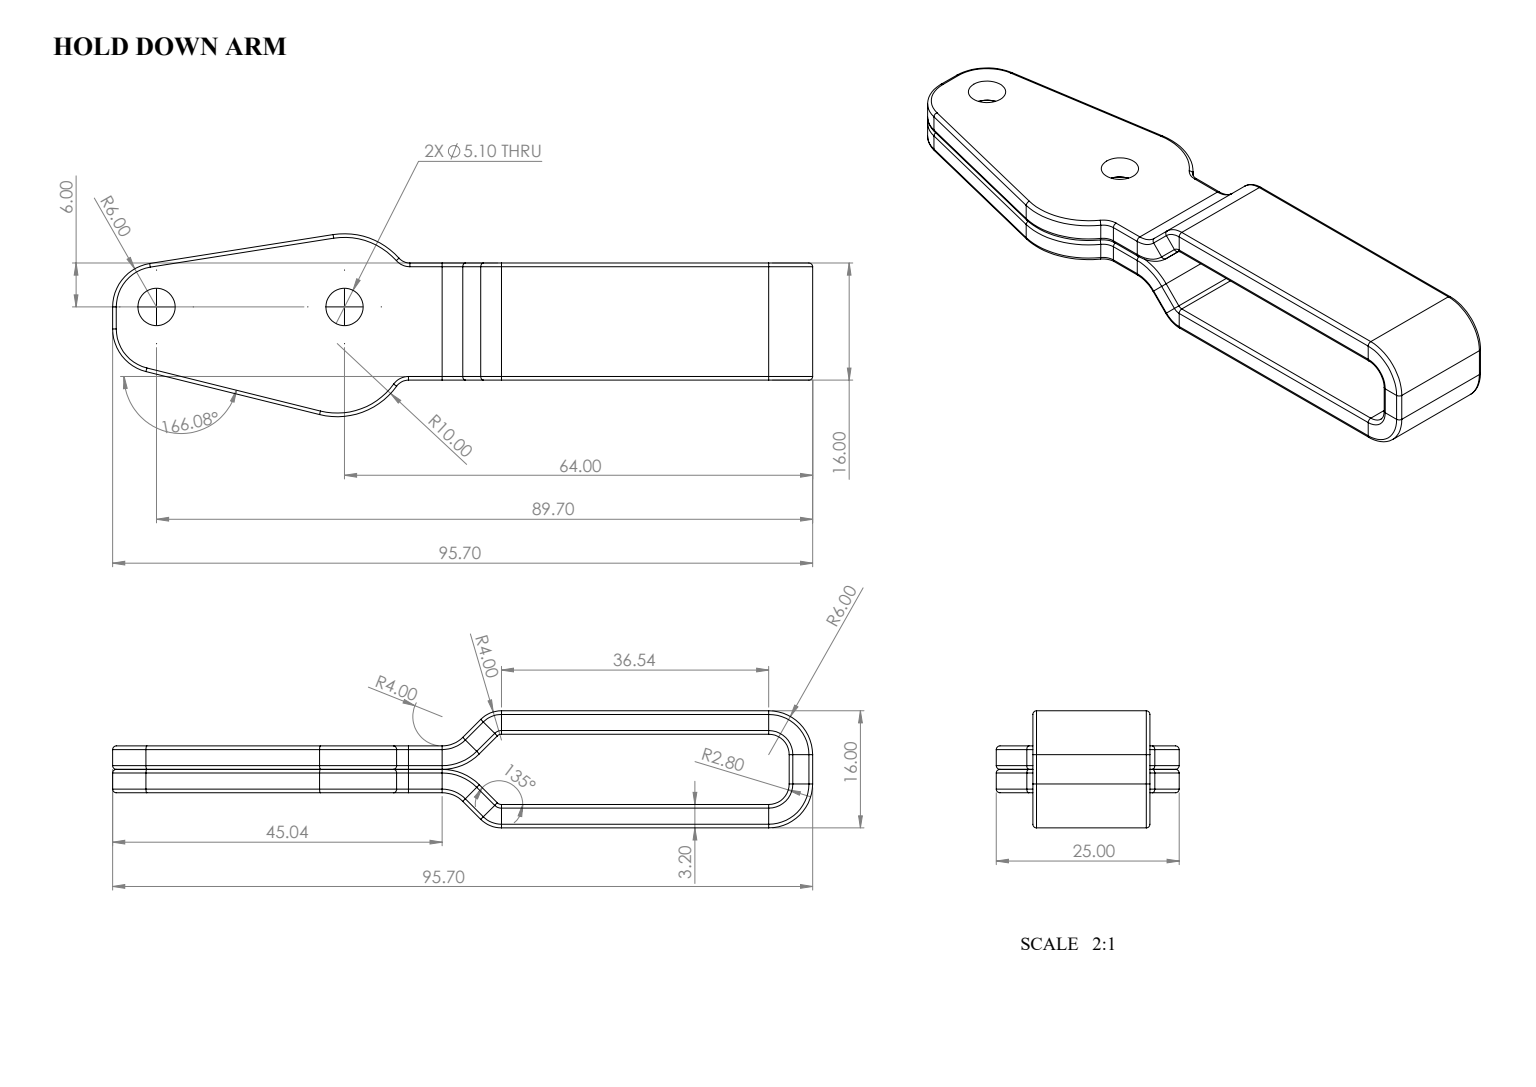
ISO-10303-21;
HEADER;
FILE_DESCRIPTION (('STEP AP214'),
    '1' );
FILE_NAME ('Hold Down Arm.step',
    '2026-10-06T08:09:25',
    ( '' ),
    ( '' ),
    'SwSTEP 2.0',
    'SolidWorks 2021',
    '' );
FILE_SCHEMA (( 'AUTOMOTIVE_DESIGN' ));
ENDSEC;

DATA;
#4=ORIENTED_EDGE ( 'NONE', *, *, #13581, .T. ) ;
#8=DIRECTION ( 'NONE',  ( 1.000000000000000000, 2.220446049250314560E-16, 0.000000000000000000 ) ) ;
#9=CARTESIAN_POINT ( 'NONE',  ( -55.05572809000119605, -2.700000000000125855, -7.500000000000062172 ) ) ;
#14=EDGE_LOOP ( 'NONE', ( #2614, #10567, #22264, #5073 ) ) ;
#18=DIRECTION ( 'NONE',  ( -1.000000000000000000, 1.424116703980815236E-16, 2.931272055834072749E-32 ) ) ;
#20=CARTESIAN_POINT ( 'NONE',  ( -47.82842712474649716, 4.371572875253824542, 8.000000000000021316 ) ) ;
#27=CARTESIAN_POINT ( 'NONE',  ( -50.65685424949274562, -3.200000000000091660, 7.500000000000076383 ) ) ;
#30=ORIENTED_EDGE ( 'NONE', *, *, #19301, .F. ) ;
#33=ORIENTED_EDGE ( 'NONE', *, *, #6783, .T. ) ;
#46=FACE_OUTER_BOUND ( 'NONE', #18970, .T. ) ;
#63=ORIENTED_EDGE ( 'NONE', *, *, #11679, .F. ) ;
#66=ORIENTED_EDGE ( 'NONE', *, *, #4342, .F. ) ;
#67=EDGE_CURVE ( 'NONE', #21664, #15682, #5815, .T. ) ;
#70=CARTESIAN_POINT ( 'NONE',  ( -42.54314575050785407, -5.300000000000037126, -7.500000000000007105 ) ) ;
#73=DIRECTION ( 'NONE',  ( -0.9878135252003118483, -1.627025617018325989E-30, 0.1556420233463095271 ) ) ;
#78=EDGE_CURVE ( 'NONE', #1099, #6825, #11430, .T. ) ;
#91=CIRCLE ( 'NONE', #20737, 0.4999999999999994449 ) ;
#92=ORIENTED_EDGE ( 'NONE', *, *, #20127, .T. ) ;
#96=DIRECTION ( 'NONE',  ( -4.336808689942052446E-15, -1.000000000000000000, -3.574525976782710619E-31 ) ) ;
#98=DIRECTION ( 'NONE',  ( 0.000000000000000000, -1.000000000000000000, 0.000000000000000000 ) ) ;
#99=DIRECTION ( 'NONE',  ( -1.000000000000000000, -2.220446049250313081E-16, 0.000000000000000000 ) ) ;
#101=ADVANCED_FACE ( 'NONE', ( #18737 ), #22509, .T. ) ;
#103=DIRECTION ( 'NONE',  ( -2.220446049250313081E-16, 1.000000000000000000, -7.025792437124636392E-31 ) ) ;
#105=LINE ( 'NONE', #16189, #2754 ) ;
#118=AXIS2_PLACEMENT_3D ( 'NONE', #12279, #12167, #17943 ) ;
#119=DIRECTION ( 'NONE',  ( -1.000000000000000000, -1.479114197289388027E-30, 2.013525853228518840E-32 ) ) ;
#121=AXIS2_PLACEMENT_3D ( 'NONE', #9275, #21645, #19978 ) ;
#122=CARTESIAN_POINT ( 'NONE',  ( -92.25000000000058265, -8.981013850637800498E-14, -2.000000000000001776 ) ) ;
#126=DIRECTION ( 'NONE',  ( 2.013525853228507892E-32, 6.902532920683810383E-31, -1.000000000000000000 ) ) ;
#128=CARTESIAN_POINT ( 'NONE',  ( -89.70000000000064233, 2.700000000000056577, -2.000000000000001776 ) ) ;
#131=CYLINDRICAL_SURFACE ( 'NONE', #16076, 2.000000000000015543 ) ;
#137=AXIS2_PLACEMENT_3D ( 'NONE', #8620, #22982, #10500 ) ;
#139=AXIS2_PLACEMENT_3D ( 'NONE', #3664, #23097, #6847 ) ;
#152=AXIS2_PLACEMENT_3D ( 'NONE', #5181, #12341, #17885 ) ;
#154=TOROIDAL_SURFACE ( 'NONE', #10279, 5.500000000000007994, 0.5000000000000000000 ) ;
#155=CARTESIAN_POINT ( 'NONE',  ( -55.25320565519145788, 0.5000000000000905942, 10.00000000000009237 ) ) ;
#156=VECTOR ( 'NONE', #8671, 1000.000000000000227 ) ;
#158=AXIS2_PLACEMENT_3D ( 'NONE', #22123, #20356, #13067 ) ;
#160=DIRECTION ( 'NONE',  ( 1.000000000000000000, 2.220446049250313081E-16, -3.656342123407315983E-48 ) ) ;
#170=AXIS2_PLACEMENT_3D ( 'NONE', #22281, #4382, #9585 ) ;
#173=VECTOR ( 'NONE', #16606, 1000.000000000000000 ) ;
#183=EDGE_CURVE ( 'NONE', #9368, #15940, #10370, .T. ) ;
#184=EDGE_CURVE ( 'NONE', #21240, #19103, #1689, .T. ) ;
#185=FACE_OUTER_BOUND ( 'NONE', #9063, .T. ) ;
#189=FACE_OUTER_BOUND ( 'NONE', #10029, .T. ) ;
#190=CARTESIAN_POINT ( 'NONE',  ( -42.54314575050778302, -8.000000000000021316, 7.500000000000034639 ) ) ;
#196=EDGE_CURVE ( 'NONE', #1099, #11721, #4693, .T. ) ;
#197=EDGE_CURVE ( 'NONE', #5639, #7574, #985, .T. ) ;
#201=AXIS2_PLACEMENT_3D ( 'NONE', #19066, #17054, #16931 ) ;
#218=AXIS2_PLACEMENT_3D ( 'NONE', #14602, #2245, #20126 ) ;
#220=DIRECTION ( 'NONE',  ( -1.000000000000000000, -2.220446049250314067E-16, 5.825996348268307008E-33 ) ) ;
#225=ORIENTED_EDGE ( 'NONE', *, *, #17691, .F. ) ;
#227=EDGE_CURVE ( 'NONE', #18640, #22996, #18594, .T. ) ;
#228=CARTESIAN_POINT ( 'NONE',  ( -55.05572809000122447, -2.700000000000125855, -10.00000000000006395 ) ) ;
#240=DIRECTION ( 'NONE',  ( -2.013525853228508439E-32, -6.779273404243028164E-31, 1.000000000000000000 ) ) ;
#242=DIRECTION ( 'NONE',  ( 1.000000000000000000, 1.479114197289387852E-30, -2.013525853228518840E-32 ) ) ;
#257=FACE_OUTER_BOUND ( 'NONE', #3493, .T. ) ;
#259=FACE_OUTER_BOUND ( 'NONE', #10192, .T. ) ;
#274=ORIENTED_EDGE ( 'NONE', *, *, #19427, .F. ) ;
#276=EDGE_LOOP ( 'NONE', ( #1805, #8526, #7103, #1700 ) ) ;
#278=VERTEX_POINT ( 'NONE', #17790 ) ;
#292=DIRECTION ( 'NONE',  ( 0.7071067811865535679, -0.7071067811865414665, 0.000000000000000000 ) ) ;
#298=CARTESIAN_POINT ( 'NONE',  ( -56.87767137932624451, -2.700000000000049472, 8.833333333333415638 ) ) ;
#302=ORIENTED_EDGE ( 'NONE', *, *, #6662, .T. ) ;
#305=CARTESIAN_POINT ( 'NONE',  ( -90.55603112840523750, -3.200000000000105427, -7.432974388601742533 ) ) ;
#307=ORIENTED_EDGE ( 'NONE', *, *, #10358, .F. ) ;
#309=ORIENTED_EDGE ( 'NONE', *, *, #10119, .F. ) ;
#310=AXIS2_PLACEMENT_3D ( 'NONE', #22356, #6236, #2234 ) ;
#311=ORIENTED_EDGE ( 'NONE', *, *, #11203, .F. ) ;
#316=LINE ( 'NONE', #16179, #14360 ) ;
#319=FACE_OUTER_BOUND ( 'NONE', #20806, .T. ) ;
#326=DIRECTION ( 'NONE',  ( 1.000000000000000000, 2.220446049250314067E-16, -5.825996348268307008E-33 ) ) ;
#329=CIRCLE ( 'NONE', #8202, 0.5000000000000004441 ) ;
#332=DIRECTION ( 'NONE',  ( 1.550910762415513985E-16, 1.000000000000000000, -8.135128085091684243E-31 ) ) ;
#333=EDGE_CURVE ( 'NONE', #15092, #15826, #3886, .T. ) ;
#336=EDGE_CURVE ( 'NONE', #17272, #9446, #19746, .T. ) ;
#369=PRODUCT_CONTEXT ( 'NONE', #23224, 'mechanical' ) ;
#377=DIRECTION ( 'NONE',  ( 0.2405376366294273427, 0.000000000000000000, -0.9706398123736372785 ) ) ;
#391=CARTESIAN_POINT ( 'NONE',  ( -0.5000000000000559552, -1.999999999999988010, -8.000000000000062172 ) ) ;
#394=EDGE_LOOP ( 'NONE', ( #15847, #9130, #15878, #21668 ) ) ;
#395=ORIENTED_EDGE ( 'NONE', *, *, #6942, .F. ) ;
#400=EDGE_LOOP ( 'NONE', ( #7462, #10799, #18667, #12854 ) ) ;
#409=DIRECTION ( 'NONE',  ( -2.220446049250313081E-16, 1.000000000000000000, -7.025792437124636392E-31 ) ) ;
#416=DIRECTION ( 'NONE',  ( 1.000000000000000000, 6.640738306473676004E-15, 4.078150875473213127E-31 ) ) ;
#425=ORIENTED_EDGE ( 'NONE', *, *, #22642, .T. ) ;
#426=EDGE_CURVE ( 'NONE', #22532, #14335, #5472, .T. ) ;
#436=CARTESIAN_POINT ( 'NONE',  ( -91.14322581977729953, 0.5000000000000073275, 6.823838874241844543 ) ) ;
#441=( LENGTH_UNIT ( ) NAMED_UNIT ( * ) SI_UNIT ( .MILLI., .METRE. ) );
#442=DIRECTION ( 'NONE',  ( -1.550910762415566494E-16, -1.000000000000000000, 8.135128085091684243E-31 ) ) ;
#454=CARTESIAN_POINT ( 'NONE',  ( -43.10883117545721888, 4.565685424949256443, -7.500000000000034639 ) ) ;
#455=FACE_OUTER_BOUND ( 'NONE', #14770, .T. ) ;
#460=CARTESIAN_POINT ( 'NONE',  ( -89.70000000000065654, 3.200000000000057021, -2.000000000000001776 ) ) ;
#461=EDGE_CURVE ( 'NONE', #6874, #3000, #20486, .T. ) ;
#472=EDGE_CURVE ( 'NONE', #1433, #3000, #8099, .T. ) ;
#474=EDGE_CURVE ( 'NONE', #5438, #4432, #6471, .T. ) ;
#477=VERTEX_POINT ( 'NONE', #15401 ) ;
#484=EDGE_CURVE ( 'NONE', #1099, #2832, #13652, .T. ) ;
#487=CYLINDRICAL_SURFACE ( 'NONE', #2237, 0.5000000000000029976 ) ;
#489=ORIENTED_EDGE ( 'NONE', *, *, #12121, .F. ) ;
#490=PLANE ( 'NONE',  #19494 ) ;
#498=CIRCLE ( 'NONE', #14398, 0.4999999999999994449 ) ;
#506=CARTESIAN_POINT ( 'NONE',  ( -42.54314575050799618, 4.799999999999998934, 8.000000000000035527 ) ) ;
#510=ORIENTED_EDGE ( 'NONE', *, *, #22197, .F. ) ;
#511=ORIENTED_EDGE ( 'NONE', *, *, #15896, .T. ) ;
#512=ORIENTED_EDGE ( 'NONE', *, *, #15274, .F. ) ;
#521=AXIS2_PLACEMENT_3D ( 'NONE', #8817, #5413, #15970 ) ;
#529=FACE_OUTER_BOUND ( 'NONE', #12268, .T. ) ;
#535=CARTESIAN_POINT ( 'NONE',  ( -89.70000000000054285, -9.020562075079396891E-14, 1.000000000000000888 ) ) ;
#544=EDGE_LOOP ( 'NONE', ( #3998, #20221, #14255, #14599 ) ) ;
#549=ADVANCED_FACE ( 'NONE', ( #5291 ), #15517, .T. ) ;
#553=AXIS2_PLACEMENT_3D ( 'NONE', #6003, #7641, #3986 ) ;
#554=FACE_OUTER_BOUND ( 'NONE', #6636, .T. ) ;
#557=EDGE_CURVE ( 'NONE', #19870, #14824, #11076, .T. ) ;
#559=CARTESIAN_POINT ( 'NONE',  ( -42.54314575050781144, -3.999999999999996447, -16.42537846091818210 ) ) ;
#565=CARTESIAN_POINT ( 'NONE',  ( -50.65685424949274562, -3.200000000000091660, 8.000000000000062172 ) ) ;
#571=ORIENTED_EDGE ( 'NONE', *, *, #22014, .F. ) ;
#576=CARTESIAN_POINT ( 'NONE',  ( -6.000000000000199840, 4.799999999999935874, 8.000000000000035527 ) ) ;
#578=DIRECTION ( 'NONE',  ( 0.7071067811865510144, 0.7071067811865441310, -9.779905552809737959E-15 ) ) ;
#586=EDGE_CURVE ( 'NONE', #15196, #6243, #21185, .T. ) ;
#600=CIRCLE ( 'NONE', #8864, 0.5000000000000028866 ) ;
#607=DIRECTION ( 'NONE',  ( 0.7071067811865502373, -0.7071067811865447972, -5.485661035786110830E-15 ) ) ;
#608=DIRECTION ( 'NONE',  ( 0.2405376366294550983, 0.000000000000000000, -0.9706398123736303951 ) ) ;
#630=ORIENTED_EDGE ( 'NONE', *, *, #14353, .F. ) ;
#653=EDGE_CURVE ( 'NONE', #19930, #15092, #3743, .T. ) ;
#658=ORIENTED_EDGE ( 'NONE', *, *, #15288, .F. ) ;
#665=AXIS2_PLACEMENT_3D ( 'NONE', #19621, #7167, #5157 ) ;
#668=CYLINDRICAL_SURFACE ( 'NONE', #15478, 0.5000000000000004441 ) ;
#671=VECTOR ( 'NONE', #10328, 1000.000000000000227 ) ;
#680=FACE_OUTER_BOUND ( 'NONE', #17185, .T. ) ;
#684=PLANE ( 'NONE',  #18357 ) ;
#691=ORIENTED_EDGE ( 'NONE', *, *, #20005, .F. ) ;
#713=CARTESIAN_POINT ( 'NONE',  ( -50.65685424949278826, 1.387778780781445676E-14, -7.500000000000034639 ) ) ;
#718=ORIENTED_EDGE ( 'NONE', *, *, #16718, .F. ) ;
#748=ORIENTED_EDGE ( 'NONE', *, *, #11622, .T. ) ;
#751=CARTESIAN_POINT ( 'NONE',  ( -49.51923881554282048, 1.137615433949801247, 7.500000000000062172 ) ) ;
#752=EDGE_CURVE ( 'NONE', #15489, #3212, #12450, .T. ) ;
#755=AXIS2_PLACEMENT_3D ( 'NONE', #13105, #409, #21706 ) ;
#756=DIRECTION ( 'NONE',  ( -1.000000000000000000, -1.479114197289388027E-30, 2.013525853228518840E-32 ) ) ;
#761=EDGE_CURVE ( 'NONE', #18638, #13378, #23145, .T. ) ;
#764=EDGE_CURVE ( 'NONE', #8174, #11574, #3261, .T. ) ;
#768=CARTESIAN_POINT ( 'NONE',  ( -95.20000000000061391, -0.5000000000000975886, 8.000000000000117240 ) ) ;
#779=EDGE_CURVE ( 'NONE', #4281, #1775, #20143, .T. ) ;
#781=ORIENTED_EDGE ( 'NONE', *, *, #14027, .T. ) ;
#786=ORIENTED_EDGE ( 'NONE', *, *, #13748, .F. ) ;
#787=DIRECTION ( 'NONE',  ( 1.000000000000000000, 1.424116703980846297E-16, -1.095779650622964657E-32 ) ) ;
#789=DIRECTION ( 'NONE',  ( 0.000000000000000000, 0.000000000000000000, 1.000000000000000000 ) ) ;
#792=DIRECTION ( 'NONE',  ( 0.9706398123736330597, 1.110223024625160485E-16, 0.2405376366294442736 ) ) ;
#798=DIRECTION ( 'NONE',  ( 1.000000000000000000, 1.479114197289387852E-30, -2.013525853228518840E-32 ) ) ;
#804=ORIENTED_EDGE ( 'NONE', *, *, #20468, .F. ) ;
#805=ORIENTED_EDGE ( 'NONE', *, *, #9969, .T. ) ;
#812=FACE_OUTER_BOUND ( 'NONE', #7748, .T. ) ;
#813=CARTESIAN_POINT ( 'NONE',  ( -45.91923881554279774, 2.462384566050190848, -7.500000000000062172 ) ) ;
#814=CARTESIAN_POINT ( 'NONE',  ( -89.70000000000057128, -0.5000000000000628386, -2.000000000000001776 ) ) ;
#817=EDGE_CURVE ( 'NONE', #5639, #8174, #15026, .T. ) ;
#830=AXIS2_PLACEMENT_3D ( 'NONE', #9486, #8070, #792 ) ;
#836=CARTESIAN_POINT ( 'NONE',  ( -95.70000000000062812, -1.318389841742373392E-13, 8.000000000000062172 ) ) ;
#837=CARTESIAN_POINT ( 'NONE',  ( -45.37157287525414517, -6.828427124746218269, 7.500000000000089706 ) ) ;
#851=CYLINDRICAL_SURFACE ( 'NONE', #5151, 0.5000000000000000000 ) ;
#852=AXIS2_PLACEMENT_3D ( 'NONE', #14679, #3854, #11035 ) ;
#853=TOROIDAL_SURFACE ( 'NONE', #8348, 3.500000000000000888, 0.5000000000000000000 ) ;
#854=EDGE_LOOP ( 'NONE', ( #1944, #11607, #22757, #20845 ) ) ;
#870=CIRCLE ( 'NONE', #1976, 0.5000000000000004441 ) ;
#873=CARTESIAN_POINT ( 'NONE',  ( -50.65685424949273141, 0.000000000000000000, 8.000000000000076383 ) ) ;
#876=( NAMED_UNIT ( * ) PLANE_ANGLE_UNIT ( ) SI_UNIT ( $, .RADIAN. ) );
#881=DIRECTION ( 'NONE',  ( -0.9878135252003118483, -1.627025617018325989E-30, 0.1556420233463091385 ) ) ;
#883=EDGE_CURVE ( 'NONE', #16517, #14933, #8878, .T. ) ;
#885=AXIS2_PLACEMENT_3D ( 'NONE', #5509, #21519, #6803 ) ;
#890=AXIS2_PLACEMENT_3D ( 'NONE', #12840, #9317, #16129 ) ;
#893=AXIS2_PLACEMENT_3D ( 'NONE', #20867, #8852, #2976 ) ;
#899=ORIENTED_EDGE ( 'NONE', *, *, #5134, .F. ) ;
#901=DIRECTION ( 'NONE',  ( 2.013525853228507892E-32, 6.902532920683810383E-31, -1.000000000000000000 ) ) ;
#929=ORIENTED_EDGE ( 'NONE', *, *, #11228, .T. ) ;
#936=DIRECTION ( 'NONE',  ( 4.336808689942052446E-15, 1.000000000000000000, 3.574525976782710619E-31 ) ) ;
#937=DIRECTION ( 'NONE',  ( 1.000000000000000000, -1.389842848855773367E-62, 2.013525853228507892E-32 ) ) ;
#939=DIRECTION ( 'NONE',  ( -1.000000000000000000, 1.550910762415508562E-16, 0.000000000000000000 ) ) ;
#943=EDGE_CURVE ( 'NONE', #17067, #4165, #11494, .T. ) ;
#959=DIRECTION ( 'NONE',  ( 1.331202777560457422E-30, 1.000000000000000000, -7.395570986446985676E-31 ) ) ;
#964=DIRECTION ( 'NONE',  ( -1.550910762415566494E-16, -1.000000000000000000, 8.135128085091684243E-31 ) ) ;
#972=FACE_OUTER_BOUND ( 'NONE', #13994, .T. ) ;
#985=LINE ( 'NONE', #6982, #17847 ) ;
#988=FACE_OUTER_BOUND ( 'NONE', #14105, .T. ) ;
#990=CARTESIAN_POINT ( 'NONE',  ( -50.65685424949267457, -7.200000000000049916, 7.500000000000047962 ) ) ;
#997=TOROIDAL_SURFACE ( 'NONE', #5495, 3.500000000000000888, 0.5000000000000000000 ) ;
#1001=CARTESIAN_POINT ( 'NONE',  ( -6.000000000000074607, -8.000000000000003553, -7.500000000000034639 ) ) ;
#1006=ORIENTED_EDGE ( 'NONE', *, *, #15901, .F. ) ;
#1014=CARTESIAN_POINT ( 'NONE',  ( -50.65685424949281668, 3.200000000000022382, 7.500000000000034639 ) ) ;
#1015=ORIENTED_EDGE ( 'NONE', *, *, #15615, .T. ) ;
#1021=DIRECTION ( 'NONE',  ( 2.220446049250313081E-16, -1.000000000000000000, 7.025792437124636392E-31 ) ) ;
#1030=CIRCLE ( 'NONE', #4015, 0.5000000000000029976 ) ;
#1041=DIRECTION ( 'NONE',  ( 1.550910762415513985E-16, 1.000000000000000000, -8.135128085091684243E-31 ) ) ;
#1051=DIRECTION ( 'NONE',  ( 1.550910762415566494E-16, 1.000000000000000000, -8.135128085091684243E-31 ) ) ;
#1054=CARTESIAN_POINT ( 'NONE',  ( -92.25000000000065370, 5.494493748869900097E-14, -2.000000000000001776 ) ) ;
#1057=CARTESIAN_POINT ( 'NONE',  ( -45.01801948466093961, 6.474873734152897242, -8.000000000000035527 ) ) ;
#1059=ADVANCED_FACE ( 'NONE', ( #812 ), #22427, .T. ) ;
#1062=CARTESIAN_POINT ( 'NONE',  ( -50.65685424949278826, 0.5000000000000213163, -7.500000000000034639 ) ) ;
#1065=AXIS2_PLACEMENT_3D ( 'NONE', #21849, #15010, #2543 ) ;
#1067=ORIENTED_EDGE ( 'NONE', *, *, #6289, .F. ) ;
#1083=STYLED_ITEM ( 'NONE', ( #20322 ), #15045 ) ;
#1088=CARTESIAN_POINT ( 'NONE',  ( -50.65685424949274562, -2.700000000000125855, 7.500000000000076383 ) ) ;
#1092=DIRECTION ( 'NONE',  ( -1.000000000000000000, -1.479114197289388027E-30, 2.013525853228518840E-32 ) ) ;
#1093=AXIS2_PLACEMENT_3D ( 'NONE', #20642, #18858, #1223 ) ;
#1099=VERTEX_POINT ( 'NONE', #13509 ) ;
#1101=EDGE_LOOP ( 'NONE', ( #16948, #7826, #13990, #15195 ) ) ;
#1107=AXIS2_PLACEMENT_3D ( 'NONE', #3565, #5092, #19911 ) ;
#1123=ADVANCED_FACE ( 'NONE', ( #22447 ), #17133, .T. ) ;
#1124=ORIENTED_EDGE ( 'NONE', *, *, #13695, .F. ) ;
#1136=VERTEX_POINT ( 'NONE', #10199 ) ;
#1151=CARTESIAN_POINT ( 'NONE',  ( -55.05572809000119605, -0.5000000000001045830, -8.000000000000090594 ) ) ;
#1152=ORIENTED_EDGE ( 'NONE', *, *, #12772, .F. ) ;
#1172=CARTESIAN_POINT ( 'NONE',  ( -42.54314575050796776, 3.999999999999996447, -8.000000000000035527 ) ) ;
#1180=ADVANCED_FACE ( 'NONE', ( #8796 ), #2504, .T. ) ;
#1182=EDGE_CURVE ( 'NONE', #6492, #18669, #10552, .T. ) ;
#1190=CIRCLE ( 'NONE', #19959, 7.200000000000046363 ) ;
#1191=CARTESIAN_POINT ( 'NONE',  ( -55.05572809000130974, 2.700000000000021938, -8.000000000000035527 ) ) ;
#1194=CARTESIAN_POINT ( 'NONE',  ( -42.54314575050792513, 3.999999999999996447, 16.42537846091821052 ) ) ;
#1204=AXIS2_PLACEMENT_3D ( 'NONE', #813, #11495, #13510 ) ;
#1205=ORIENTED_EDGE ( 'NONE', *, *, #8263, .F. ) ;
#1216=DIRECTION ( 'NONE',  ( -1.000000000000000000, 6.938893903907186568E-15, 0.000000000000000000 ) ) ;
#1220=CARTESIAN_POINT ( 'NONE',  ( -91.14322581977729953, 2.700000000000014833, 6.823838874241844543 ) ) ;
#1223=DIRECTION ( 'NONE',  ( -1.000000000000000000, -1.144237745222090235E-17, 1.939787525279694125E-32 ) ) ;
#1224=VECTOR ( 'NONE', #17612, 1000.000000000000114 ) ;
#1225=DIRECTION ( 'NONE',  ( 0.1556420233463076119, 0.000000000000000000, 0.9878135252003121813 ) ) ;
#1226=AXIS2_PLACEMENT_3D ( 'NONE', #7718, #9254, #20081 ) ;
#1237=EDGE_CURVE ( 'NONE', #4862, #16835, #16732, .T. ) ;
#1239=ORIENTED_EDGE ( 'NONE', *, *, #2920, .T. ) ;
#1240=AXIS2_PLACEMENT_3D ( 'NONE', #7811, #18512, #20522 ) ;
#1241=AXIS2_PLACEMENT_3D ( 'NONE', #1247, #17337, #14055 ) ;
#1242=CIRCLE ( 'NONE', #11361, 0.5000000000000029976 ) ;
#1247=CARTESIAN_POINT ( 'NONE',  ( -42.54314575050785407, -4.000000000000034639, -7.500000000000007105 ) ) ;
#1249=CARTESIAN_POINT ( 'NONE',  ( -50.65685424949263904, -7.200000000000071232, -7.500000000000034639 ) ) ;
#1250=CARTESIAN_POINT ( 'NONE',  ( -1.110223024625156540E-13, -1.999999999999988010, 7.500000000000020428 ) ) ;
#1259=VECTOR ( 'NONE', #901, 1000.000000000000000 ) ;
#1270=ORIENTED_EDGE ( 'NONE', *, *, #20922, .F. ) ;
#1274=AXIS2_PLACEMENT_3D ( 'NONE', #6348, #13400, #4804 ) ;
#1289=FACE_OUTER_BOUND ( 'NONE', #19754, .T. ) ;
#1291=DIRECTION ( 'NONE',  ( -2.013525853228507892E-32, -6.902532920683810383E-31, 1.000000000000000000 ) ) ;
#1292=AXIS2_PLACEMENT_3D ( 'NONE', #17237, #11834, #13607 ) ;
#1301=DIRECTION ( 'NONE',  ( -1.550910762415566494E-16, -1.000000000000000000, 8.135128085091684243E-31 ) ) ;
#1304=AXIS2_PLACEMENT_3D ( 'NONE', #16015, #18033, #160 ) ;
#1307=LINE ( 'NONE', #9688, #8776 ) ;
#1309=CARTESIAN_POINT ( 'NONE',  ( -49.51923881554282048, 1.137615433949801247, 8.000000000000062172 ) ) ;
#1310=CARTESIAN_POINT ( 'NONE',  ( -95.70000000000071338, 2.775557561562891351E-14, 1.000000000000070166 ) ) ;
#1313=ADVANCED_FACE ( 'NONE', ( #988 ), #13453, .T. ) ;
#1314=CARTESIAN_POINT ( 'NONE',  ( -87.15000000000064517, 5.607736497381665307E-14, -2.000000000000001332 ) ) ;
#1318=ADVANCED_FACE ( 'NONE', ( #17075 ), #22512, .F. ) ;
#1320=LINE ( 'NONE', #19072, #6700 ) ;
#1321=EDGE_CURVE ( 'NONE', #5639, #8147, #17136, .T. ) ;
#1329=VERTEX_POINT ( 'NONE', #16847 ) ;
#1333=DIRECTION ( 'NONE',  ( -1.144237745221811361E-17, 1.000000000000000000, -7.025792437124636392E-31 ) ) ;
#1338=CARTESIAN_POINT ( 'NONE',  ( -6.000000000000143885, -2.000000000000043521, -8.000000000000035527 ) ) ;
#1339=EDGE_CURVE ( 'NONE', #8929, #15576, #4500, .T. ) ;
#1346=DIRECTION ( 'NONE',  ( 0.000000000000000000, 0.000000000000000000, -1.000000000000000000 ) ) ;
#1348=DIRECTION ( 'NONE',  ( 2.220446049250313081E-16, -1.000000000000000000, 7.025792437124636392E-31 ) ) ;
#1349=CARTESIAN_POINT ( 'NONE',  ( -50.65685424949274562, 0.5000000000000143219, -8.000000000000062172 ) ) ;
#1352=ORIENTED_EDGE ( 'NONE', *, *, #22036, .T. ) ;
#1355=EDGE_LOOP ( 'NONE', ( #9247, #2066, #15136, #15479 ) ) ;
#1374=EDGE_CURVE ( 'NONE', #6466, #18914, #19429, .T. ) ;
#1382=EDGE_LOOP ( 'NONE', ( #8989, #21213, #23151, #14355 ) ) ;
#1383=ORIENTED_EDGE ( 'NONE', *, *, #22635, .F. ) ;
#1384=ORIENTED_EDGE ( 'NONE', *, *, #18533, .F. ) ;
#1386=LINE ( 'NONE', #22918, #16285 ) ;
#1396=TOROIDAL_SURFACE ( 'NONE', #14920, 1.300000000000000711, 0.5000000000000000000 ) ;
#1401=ORIENTED_EDGE ( 'NONE', *, *, #12037, .T. ) ;
#1402=ORIENTED_EDGE ( 'NONE', *, *, #14002, .F. ) ;
#1414=CARTESIAN_POINT ( 'NONE',  ( -64.00000000000045475, 6.245004513516505540E-14, -1.999999999999974021 ) ) ;
#1415=DIRECTION ( 'NONE',  ( -1.331202777560457422E-30, -1.000000000000000000, 7.395570986446985676E-31 ) ) ;
#1418=CIRCLE ( 'NONE', #13068, 2.550000000000010481 ) ;
#1422=DIRECTION ( 'NONE',  ( -2.013525853228507892E-32, -6.902532920683810383E-31, 1.000000000000000000 ) ) ;
#1424=CARTESIAN_POINT ( 'NONE',  ( -50.65685424949280247, 1.387778780781445676E-14, 8.000000000000090594 ) ) ;
#1428=AXIS2_PLACEMENT_3D ( 'NONE', #13780, #1092, #17412 ) ;
#1433=VERTEX_POINT ( 'NONE', #6398 ) ;
#1442=DIRECTION ( 'NONE',  ( -2.220446049250313081E-16, 1.000000000000000000, -7.025792437124636392E-31 ) ) ;
#1444=VECTOR ( 'NONE', #442, 1000.000000000000000 ) ;
#1454=ORIENTED_EDGE ( 'NONE', *, *, #13692, .F. ) ;
#1456=ORIENTED_EDGE ( 'NONE', *, *, #16684, .T. ) ;
#1458=EDGE_CURVE ( 'NONE', #4755, #10141, #22619, .T. ) ;
#1464=ORIENTED_EDGE ( 'NONE', *, *, #21499, .F. ) ;
#1470=CARTESIAN_POINT ( 'NONE',  ( -64.00000000000038369, -3.200000000000081446, -2.000000000000029310 ) ) ;
#1471=EDGE_CURVE ( 'NONE', #21722, #18197, #11793, .T. ) ;
#1482=AXIS2_PLACEMENT_3D ( 'NONE', #12903, #16644, #3954 ) ;
#1486=ORIENTED_EDGE ( 'NONE', *, *, #426, .F. ) ;
#1490=CARTESIAN_POINT ( 'NONE',  ( -89.70000000000055707, -3.200000000000105427, -1.999999999999946265 ) ) ;
#1506=CARTESIAN_POINT ( 'NONE',  ( -2.700000000000119194, 1.999999999999967137, -8.000000000000007105 ) ) ;
#1508=AXIS2_PLACEMENT_3D ( 'NONE', #5115, #8531, #3590 ) ;
#1519=TOROIDAL_SURFACE ( 'NONE', #21814, 6.700000000000001066, 0.5000000000000000000 ) ;
#1521=ORIENTED_EDGE ( 'NONE', *, *, #13820, .F. ) ;
#1524=EDGE_LOOP ( 'NONE', ( #1663, #9843, #66, #6122 ) ) ;
#1525=ORIENTED_EDGE ( 'NONE', *, *, #5225, .T. ) ;
#1532=FACE_OUTER_BOUND ( 'NONE', #21083, .T. ) ;
#1533=DIRECTION ( 'NONE',  ( 1.000000000000000000, 0.000000000000000000, 0.000000000000000000 ) ) ;
#1539=DIRECTION ( 'NONE',  ( 2.013525853228507892E-32, 6.902532920683810383E-31, -1.000000000000000000 ) ) ;
#1551=CARTESIAN_POINT ( 'NONE',  ( -89.70000000000064233, 5.551115123125782702E-14, -2.000000000000001776 ) ) ;
#1552=DIRECTION ( 'NONE',  ( 1.331202777560457422E-30, 1.000000000000000000, -7.395570986446985676E-31 ) ) ;
#1555=CARTESIAN_POINT ( 'NONE',  ( -47.47487373415324186, 4.018019484660559471, 8.000000000000062172 ) ) ;
#1557=DIRECTION ( 'NONE',  ( -1.550910762415566494E-16, -1.000000000000000000, 8.135128085091684243E-31 ) ) ;
#1564=DIRECTION ( 'NONE',  ( 0.000000000000000000, 0.000000000000000000, 1.000000000000000000 ) ) ;
#1575=AXIS2_PLACEMENT_3D ( 'NONE', #22054, #20406, #22400 ) ;
#1588=CYLINDRICAL_SURFACE ( 'NONE', #22687, 2.550000000000010481 ) ;
#1589=LINE ( 'NONE', #13077, #14723 ) ;
#1595=CYLINDRICAL_SURFACE ( 'NONE', #10383, 0.5000000000000000000 ) ;
#1596=ORIENTED_EDGE ( 'NONE', *, *, #20698, .F. ) ;
#1599=LINE ( 'NONE', #16169, #12664 ) ;
#1603=EDGE_LOOP ( 'NONE', ( #13242, #14531, #7061, #6609 ) ) ;
#1612=DIRECTION ( 'NONE',  ( 1.550910762415566494E-16, 1.000000000000000000, -8.135128085091684243E-31 ) ) ;
#1616=ADVANCED_FACE ( 'NONE', ( #19674 ), #7208, .T. ) ;
#1620=VECTOR ( 'NONE', #8184, 1000.000000000000000 ) ;
#1631=ORIENTED_EDGE ( 'NONE', *, *, #653, .F. ) ;
#1632=EDGE_CURVE ( 'NONE', #15165, #21891, #10736, .T. ) ;
#1635=ORIENTED_EDGE ( 'NONE', *, *, #1374, .F. ) ;
#1641=ORIENTED_EDGE ( 'NONE', *, *, #10677, .T. ) ;
#1645=EDGE_CURVE ( 'NONE', #10770, #2913, #600, .T. ) ;
#1650=DIRECTION ( 'NONE',  ( 2.013525853228508439E-32, 6.779273404243028164E-31, -1.000000000000000000 ) ) ;
#1661=DIRECTION ( 'NONE',  ( 1.000000000000000000, 1.479114197289388027E-30, -2.013525853228518840E-32 ) ) ;
#1663=ORIENTED_EDGE ( 'NONE', *, *, #15877, .T. ) ;
#1672=CARTESIAN_POINT ( 'NONE',  ( -67.28510754798018922, 1.387778780781445676E-14, 12.22107821754958579 ) ) ;
#1682=DIRECTION ( 'NONE',  ( 1.387778780781437314E-14, 0.000000000000000000, -1.000000000000000000 ) ) ;
#1684=DIRECTION ( 'NONE',  ( -2.013525853228507892E-32, -6.902532920683810383E-31, 1.000000000000000000 ) ) ;
#1689=CIRCLE ( 'NONE', #7335, 0.5000000000000019984 ) ;
#1693=EDGE_CURVE ( 'NONE', #10146, #11081, #6719, .T. ) ;
#1694=VERTEX_POINT ( 'NONE', #16697 ) ;
#1700=ORIENTED_EDGE ( 'NONE', *, *, #333, .T. ) ;
#1702=ORIENTED_EDGE ( 'NONE', *, *, #17416, .F. ) ;
#1714=CARTESIAN_POINT ( 'NONE',  ( -50.65685424949262483, -7.200000000000071232, -16.89924331519437928 ) ) ;
#1717=DIRECTION ( 'NONE',  ( 1.000000000000000000, -1.365024226554777796E-62, 2.013525853228508713E-32 ) ) ;
#1719=ORIENTED_EDGE ( 'NONE', *, *, #2803, .T. ) ;
#1728=CYLINDRICAL_SURFACE ( 'NONE', #12093, 0.5000000000000004441 ) ;
#1729=CARTESIAN_POINT ( 'NONE',  ( -50.65685424949281668, 1.387778780781445676E-14, 7.500000000000034639 ) ) ;
#1733=LINE ( 'NONE', #14216, #14846 ) ;
#1736=CARTESIAN_POINT ( 'NONE',  ( -90.63385214007844581, 2.700000000000056577, -7.926881151201908615 ) ) ;
#1738=AXIS2_PLACEMENT_3D ( 'NONE', #18433, #332, #9267 ) ;
#1743=VERTEX_POINT ( 'NONE', #11295 ) ;
#1756=DIRECTION ( 'NONE',  ( 2.013525853228507892E-32, 6.902532920683810383E-31, -1.000000000000000000 ) ) ;
#1757=EDGE_CURVE ( 'NONE', #11721, #1694, #2590, .T. ) ;
#1763=CARTESIAN_POINT ( 'NONE',  ( -64.00000000000045475, 0.5000000000000490719, -1.999999999999974021 ) ) ;
#1766=CARTESIAN_POINT ( 'NONE',  ( -65.00000000000044054, -2.700000000000084110, 2.999999999999947153 ) ) ;
#1767=ADVANCED_FACE ( 'NONE', ( #5897 ), #490, .T. ) ;
#1768=ORIENTED_EDGE ( 'NONE', *, *, #752, .T. ) ;
#1770=EDGE_CURVE ( 'NONE', #7684, #10125, #13996, .T. ) ;
#1771=EDGE_CURVE ( 'NONE', #22415, #2139, #22955, .T. ) ;
#1775=VERTEX_POINT ( 'NONE', #12217 ) ;
#1781=DIRECTION ( 'NONE',  ( -3.469446951953634699E-15, 1.000000000000000000, -4.336808689942038246E-15 ) ) ;
#1783=EDGE_CURVE ( 'NONE', #11087, #21212, #20847, .T. ) ;
#1785=AXIS2_PLACEMENT_3D ( 'NONE', #21770, #12462, #242 ) ;
#1790=CARTESIAN_POINT ( 'NONE',  ( -55.05572809000126711, 0.5000000000000143219, -7.500000000000034639 ) ) ;
#1792=DIRECTION ( 'NONE',  ( -2.013525853228507892E-32, -6.902532920683810383E-31, 1.000000000000000000 ) ) ;
#1794=AXIS2_PLACEMENT_3D ( 'NONE', #17282, #15404, #6475 ) ;
#1801=ORIENTED_EDGE ( 'NONE', *, *, #3375, .T. ) ;
#1803=ORIENTED_EDGE ( 'NONE', *, *, #18662, .T. ) ;
#1805=ORIENTED_EDGE ( 'NONE', *, *, #4040, .F. ) ;
#1810=EDGE_CURVE ( 'NONE', #5384, #15489, #6597, .T. ) ;
#1816=DIRECTION ( 'NONE',  ( 0.7071067811865718866, 0.7071067811865232589, 0.000000000000000000 ) ) ;
#1818=EDGE_CURVE ( 'NONE', #7626, #21952, #22831, .T. ) ;
#1830=CARTESIAN_POINT ( 'NONE',  ( -57.28378781035996070, -2.700000000000049472, 8.541666666666781538 ) ) ;
#1831=ORIENTED_EDGE ( 'NONE', *, *, #764, .T. ) ;
#1841=DIRECTION ( 'NONE',  ( -2.220446049250313081E-16, 1.000000000000000000, -7.025792437124636392E-31 ) ) ;
#1844=DIRECTION ( 'NONE',  ( 0.000000000000000000, -1.000000000000000000, 0.000000000000000000 ) ) ;
#1848=CARTESIAN_POINT ( 'NONE',  ( -47.82842712474641189, -4.371572875253862733, 7.500000000000047962 ) ) ;
#1853=FACE_OUTER_BOUND ( 'NONE', #7005, .T. ) ;
#1866=CARTESIAN_POINT ( 'NONE',  ( -6.000000000000074607, 1.999999999999960032, 7.500000000000062172 ) ) ;
#1868=CARTESIAN_POINT ( 'NONE',  ( -43.10883117545713361, 4.565685424949256443, 8.000000000000035527 ) ) ;
#1869=DIRECTION ( 'NONE',  ( 1.000000000000000000, -1.389842848855773583E-62, 2.013525853228507892E-32 ) ) ;
#1874=DIRECTION ( 'NONE',  ( 0.000000000000000000, 0.000000000000000000, -1.000000000000000000 ) ) ;
#1880=VERTEX_POINT ( 'NONE', #10126 ) ;
#1883=VERTEX_POINT ( 'NONE', #6713 ) ;
#1884=ORIENTED_EDGE ( 'NONE', *, *, #13567, .T. ) ;
#1904=EDGE_CURVE ( 'NONE', #16829, #13948, #12688, .T. ) ;
#1905=DIRECTION ( 'NONE',  ( -0.7071067811865485719, 0.7071067811865464625, 1.010793663541191362E-16 ) ) ;
#1910=VERTEX_POINT ( 'NONE', #1191 ) ;
#1919=VERTEX_POINT ( 'NONE', #6956 ) ;
#1923=FACE_OUTER_BOUND ( 'NONE', #21813, .T. ) ;
#1925=DIRECTION ( 'NONE',  ( 2.220446049250313081E-16, -1.000000000000000000, 7.025792437124636392E-31 ) ) ;
#1936=FACE_OUTER_BOUND ( 'NONE', #20385, .T. ) ;
#1943=EDGE_LOOP ( 'NONE', ( #17781, #12744, #2271, #11404 ) ) ;
#1944=ORIENTED_EDGE ( 'NONE', *, *, #21206, .T. ) ;
#1959=EDGE_CURVE ( 'NONE', #15940, #5921, #19878, .T. ) ;
#1962=VECTOR ( 'NONE', #19867, 1000.000000000000114 ) ;
#1964=FACE_OUTER_BOUND ( 'NONE', #13440, .T. ) ;
#1970=DIRECTION ( 'NONE',  ( 1.550910762415566494E-16, 1.000000000000000000, -8.135128085091684243E-31 ) ) ;
#1971=FACE_OUTER_BOUND ( 'NONE', #6649, .T. ) ;
#1976=AXIS2_PLACEMENT_3D ( 'NONE', #10040, #22166, #20755 ) ;
#1979=EDGE_CURVE ( 'NONE', #8147, #2421, #17962, .T. ) ;
#1980=AXIS2_PLACEMENT_3D ( 'NONE', #4434, #15487, #15248 ) ;
#1994=AXIS2_PLACEMENT_3D ( 'NONE', #1866, #1650, #5061 ) ;
#1996=AXIS2_PLACEMENT_3D ( 'NONE', #15198, #4731, #13791 ) ;
#1998=ORIENTED_EDGE ( 'NONE', *, *, #5798, .T. ) ;
#2005=DIRECTION ( 'NONE',  ( -0.7071067811865485719, 0.7071067811865464625, 1.010793663541191485E-16 ) ) ;
#2018=DIRECTION ( 'NONE',  ( 0.7071067811865485719, -0.7071067811865463515, -1.010793663541191485E-16 ) ) ;
#2019=DIRECTION ( 'NONE',  ( 0.7071067811865464625, 0.7071067811865486830, 2.121016688166348642E-16 ) ) ;
#2028=CIRCLE ( 'NONE', #11046, 2.550000000000010481 ) ;
#2034=EDGE_CURVE ( 'NONE', #10886, #5077, #2545, .T. ) ;
#2037=ORIENTED_EDGE ( 'NONE', *, *, #20019, .F. ) ;
#2044=LINE ( 'NONE', #9111, #6756 ) ;
#2053=DIRECTION ( 'NONE',  ( -0.9878135252003127365, -2.193386639427060722E-16, 0.1556420233463029767 ) ) ;
#2055=EDGE_LOOP ( 'NONE', ( #1464, #14627, #10245, #18618 ) ) ;
#2061=ORIENTED_EDGE ( 'NONE', *, *, #9969, .F. ) ;
#2066=ORIENTED_EDGE ( 'NONE', *, *, #20495, .F. ) ;
#2081=CARTESIAN_POINT ( 'NONE',  ( -45.01801948466087566, 6.474873734152869709, 8.000000000000007105 ) ) ;
#2083=DIRECTION ( 'NONE',  ( -1.000000000000000000, 1.389842848855773151E-62, -2.013525853228507618E-32 ) ) ;
#2092=EDGE_CURVE ( 'NONE', #17188, #8087, #7809, .T. ) ;
#2097=VERTEX_POINT ( 'NONE', #7522 ) ;
#2100=CARTESIAN_POINT ( 'NONE',  ( -43.46238456605036760, -4.919238815542504639, -8.000000000000062172 ) ) ;
#2102=EDGE_CURVE ( 'NONE', #13536, #6998, #4419, .T. ) ;
#2103=DIRECTION ( 'NONE',  ( 1.000000000000000000, 0.000000000000000000, 0.000000000000000000 ) ) ;
#2104=VECTOR ( 'NONE', #1291, 1000.000000000000000 ) ;
#2105=CARTESIAN_POINT ( 'NONE',  ( -55.25320565519152893, 1.040834085586084257E-13, 8.000000000000035527 ) ) ;
#2111=AXIS2_PLACEMENT_3D ( 'NONE', #17977, #12552, #1844 ) ;
#2113=ORIENTED_EDGE ( 'NONE', *, *, #461, .F. ) ;
#2118=AXIS2_PLACEMENT_3D ( 'NONE', #12144, #15902, #14155 ) ;
#2119=CARTESIAN_POINT ( 'NONE',  ( -3.200000000000091660, -6.938893903907228378E-14, 8.000000000000035527 ) ) ;
#2123=DIRECTION ( 'NONE',  ( 1.000000000000000000, 1.424116703980846297E-16, -1.095779650622964657E-32 ) ) ;
#2125=DIRECTION ( 'NONE',  ( 0.000000000000000000, 1.000000000000000000, 0.000000000000000000 ) ) ;
#2126=CARTESIAN_POINT ( 'NONE',  ( -50.65685424949274562, -2.700000000000125855, 8.000000000000062172 ) ) ;
#2139=VERTEX_POINT ( 'NONE', #2100 ) ;
#2144=ORIENTED_EDGE ( 'NONE', *, *, #5082, .F. ) ;
#2154=CYLINDRICAL_SURFACE ( 'NONE', #15549, 4.000000000000023981 ) ;
#2170=LINE ( 'NONE', #3707, #22791 ) ;
#2179=VECTOR ( 'NONE', #21168, 1000.000000000000000 ) ;
#2190=CARTESIAN_POINT ( 'NONE',  ( -6.000000000000047073, -4.800000000000006040, 8.000000000000090594 ) ) ;
#2191=CARTESIAN_POINT ( 'NONE',  ( -45.56568542494955665, 0.5000000000000559552, -8.000000000000062172 ) ) ;
#2201=VECTOR ( 'NONE', #15333, 1000.000000000000114 ) ;
#2207=EDGE_CURVE ( 'NONE', #13979, #2913, #6107, .T. ) ;
#2220=CARTESIAN_POINT ( 'NONE',  ( -45.56568542494949980, -2.108831175456918228, -7.500000000000007105 ) ) ;
#2233=AXIS2_PLACEMENT_3D ( 'NONE', #1790, #10945, #16126 ) ;
#2234=DIRECTION ( 'NONE',  ( 1.000000000000000000, 2.365532012695631919E-16, -4.455085290576773719E-15 ) ) ;
#2237=AXIS2_PLACEMENT_3D ( 'NONE', #17046, #959, #8123 ) ;
#2245=DIRECTION ( 'NONE',  ( 1.550910762415566494E-16, 1.000000000000000000, -8.135128085091684243E-31 ) ) ;
#2248=DIRECTION ( 'NONE',  ( 2.013525853228508439E-32, 6.779273404243028164E-31, -1.000000000000000000 ) ) ;
#2251=DIRECTION ( 'NONE',  ( -1.000000000000000000, 1.389842848855773367E-62, -2.013525853228507892E-32 ) ) ;
#2267=ADVANCED_FACE ( 'NONE', ( #8566 ), #22923, .T. ) ;
#2271=ORIENTED_EDGE ( 'NONE', *, *, #5661, .F. ) ;
#2277=ORIENTED_EDGE ( 'NONE', *, *, #12230, .T. ) ;
#2278=DIRECTION ( 'NONE',  ( -2.220446049250313081E-16, 1.000000000000000000, -7.025792437124636392E-31 ) ) ;
#2279=DIRECTION ( 'NONE',  ( 2.013525853228507892E-32, 6.902532920683810383E-31, -1.000000000000000000 ) ) ;
#2280=CARTESIAN_POINT ( 'NONE',  ( -6.000000000000088818, 7.499999999999958256, 8.000000000000035527 ) ) ;
#2295=ORIENTED_EDGE ( 'NONE', *, *, #10778, .F. ) ;
#2296=CARTESIAN_POINT ( 'NONE',  ( -91.02295700146262902, 6.938893903907228378E-15, 6.338518968055040226 ) ) ;
#2308=DIRECTION ( 'NONE',  ( -2.013525853219289976E-32, 5.941108692445745160E-30, 1.000000000000000000 ) ) ;
#2315=CARTESIAN_POINT ( 'NONE',  ( -50.65685424949275983, -0.5000000000000905942, -8.000000000000007105 ) ) ;
#2318=CIRCLE ( 'NONE', #17336, 0.4999999999999994449 ) ;
#2334=CARTESIAN_POINT ( 'NONE',  ( -6.000000000000088818, 7.999999999999958256, 8.000000000000035527 ) ) ;
#2346=ORIENTED_EDGE ( 'NONE', *, *, #1783, .F. ) ;
#2348=AXIS2_PLACEMENT_3D ( 'NONE', #21126, #14297, #4995 ) ;
#2351=ADVANCED_FACE ( 'NONE', ( #23040 ), #7160, .F. ) ;
#2354=CARTESIAN_POINT ( 'NONE',  ( -6.000000000000143885, 1.999999999999960032, 8.000000000000062172 ) ) ;
#2359=EDGE_CURVE ( 'NONE', #6825, #16331, #3277, .T. ) ;
#2368=AXIS2_PLACEMENT_3D ( 'NONE', #16983, #8064, #20665 ) ;
#2372=CARTESIAN_POINT ( 'NONE',  ( -50.65685424949270299, 7.200000000000025935, 7.500000000000062172 ) ) ;
#2390=ORIENTED_EDGE ( 'NONE', *, *, #3134, .T. ) ;
#2393=CIRCLE ( 'NONE', #14786, 0.5000000000000028866 ) ;
#2394=DIRECTION ( 'NONE',  ( -2.013525853228507892E-32, -6.902532920683810383E-31, 1.000000000000000000 ) ) ;
#2396=EDGE_CURVE ( 'NONE', #9669, #13984, #2561, .T. ) ;
#2397=FACE_OUTER_BOUND ( 'NONE', #21427, .T. ) ;
#2402=CARTESIAN_POINT ( 'NONE',  ( -95.20000000000055707, -3.200000000000064126, -2.000000000000001776 ) ) ;
#2411=ORIENTED_EDGE ( 'NONE', *, *, #17578, .F. ) ;
#2418=AXIS2_PLACEMENT_3D ( 'NONE', #11665, #18848, #11556 ) ;
#2421=VERTEX_POINT ( 'NONE', #8913 ) ;
#2422=LINE ( 'NONE', #16521, #22628 ) ;
#2424=CARTESIAN_POINT ( 'NONE',  ( -57.28378781036000333, 0.5000000000000905942, 8.541666666666698049 ) ) ;
#2434=SURFACE_STYLE_USAGE ( .BOTH. , #18325 ) ;
#2441=ORIENTED_EDGE ( 'NONE', *, *, #16109, .T. ) ;
#2443=LINE ( 'NONE', #4678, #6493 ) ;
#2446=FACE_OUTER_BOUND ( 'NONE', #4526, .T. ) ;
#2448=CARTESIAN_POINT ( 'NONE',  ( -6.000000000000074607, 1.999999999999960032, 7.500000000000062172 ) ) ;
#2456=CARTESIAN_POINT ( 'NONE',  ( -50.65685424949267457, -7.200000000000049916, 7.500000000000047962 ) ) ;
#2459=EDGE_CURVE ( 'NONE', #19105, #20271, #10443, .T. ) ;
#2468=ADVANCED_FACE ( 'NONE', ( #9029 ), #15359, .T. ) ;
#2474=DIRECTION ( 'NONE',  ( 0.1556420233463076119, 0.000000000000000000, 0.9878135252003121813 ) ) ;
#2482=ADVANCED_FACE ( 'NONE', ( #12312 ), #17616, .T. ) ;
#2488=DIRECTION ( 'NONE',  ( -0.6666666666666649643, -4.683861624749726065E-31, -0.7453559924999314523 ) ) ;
#2502=DIRECTION ( 'NONE',  ( 1.000000000000000000, 1.479114197289388027E-30, -2.013525853228518840E-32 ) ) ;
#2504=TOROIDAL_SURFACE ( 'NONE', #11151, 1.300000000000000711, 0.5000000000000000000 ) ;
#2505=DIRECTION ( 'NONE',  ( 0.000000000000000000, 1.000000000000000000, 0.000000000000000000 ) ) ;
#2509=VECTOR ( 'NONE', #13919, 1000.000000000000000 ) ;
#2513=AXIS2_PLACEMENT_3D ( 'NONE', #14721, #9085, #20142 ) ;
#2517=DIRECTION ( 'NONE',  ( 0.1556420233463076119, 0.000000000000000000, 0.9878135252003121813 ) ) ;
#2522=EDGE_CURVE ( 'NONE', #11952, #11922, #5989, .T. ) ;
#2523=AXIS2_PLACEMENT_3D ( 'NONE', #1490, #14193, #6906 ) ;
#2529=ADVANCED_FACE ( 'NONE', ( #18654 ), #11011, .T. ) ;
#2533=ORIENTED_EDGE ( 'NONE', *, *, #15752, .F. ) ;
#2537=DIRECTION ( 'NONE',  ( -0.8122328620674128530, 0.000000000000000000, -0.5833333333333344806 ) ) ;
#2543=DIRECTION ( 'NONE',  ( -1.000000000000000000, 1.389842848855773367E-62, -2.013525853228507892E-32 ) ) ;
#2545=CIRCLE ( 'NONE', #6686, 1.300000000000009592 ) ;
#2548=( NAMED_UNIT ( * ) SI_UNIT ( $, .STERADIAN. ) SOLID_ANGLE_UNIT ( ) );
#2561=CIRCLE ( 'NONE', #20610, 3.300000000000020250 ) ;
#2562=CARTESIAN_POINT ( 'NONE',  ( -95.70000000000059970, -2.700000000000119194, -2.000000000000029310 ) ) ;
#2563=DIRECTION ( 'NONE',  ( 1.550910762415566494E-16, 1.000000000000000000, -8.135128085091684243E-31 ) ) ;
#2565=CIRCLE ( 'NONE', #15708, 10.00000000000006395 ) ;
#2573=DIRECTION ( 'NONE',  ( -2.013525853228507892E-32, -6.902532920683810383E-31, 1.000000000000000000 ) ) ;
#2574=CARTESIAN_POINT ( 'NONE',  ( -64.00000000000038369, -2.700000000000091216, -2.000000000000029310 ) ) ;
#2579=ORIENTED_EDGE ( 'NONE', *, *, #4422, .T. ) ;
#2580=AXIS2_PLACEMENT_3D ( 'NONE', #9270, #9616, #22204 ) ;
#2581=AXIS2_PLACEMENT_3D ( 'NONE', #11941, #4662, #22426 ) ;
#2583=ORIENTED_EDGE ( 'NONE', *, *, #2663, .F. ) ;
#2584=ORIENTED_EDGE ( 'NONE', *, *, #1979, .T. ) ;
#2587=DIRECTION ( 'NONE',  ( -1.550910762415566494E-16, -1.000000000000000000, 8.135128085091684243E-31 ) ) ;
#2588=FACE_OUTER_BOUND ( 'NONE', #14280, .T. ) ;
#2590=LINE ( 'NONE', #9772, #8971 ) ;
#2591=DIRECTION ( 'NONE',  ( -1.000000000000000000, -1.387778780781438734E-14, -1.404432126150815135E-14 ) ) ;
#2592=DIRECTION ( 'NONE',  ( 1.000000000000000000, 2.220446049250313081E-16, -3.656342123407315983E-48 ) ) ;
#2601=EDGE_CURVE ( 'NONE', #15092, #2139, #8615, .T. ) ;
#2603=CARTESIAN_POINT ( 'NONE',  ( -95.20000000000065654, 6.938893903907228378E-15, 1.000000000000042633 ) ) ;
#2604=CIRCLE ( 'NONE', #19520, 9.500000000000056843 ) ;
#2607=CARTESIAN_POINT ( 'NONE',  ( -95.20000000000065654, 3.200000000000015277, 1.000000000000042633 ) ) ;
#2613=ORIENTED_EDGE ( 'NONE', *, *, #6350, .F. ) ;
#2614=ORIENTED_EDGE ( 'NONE', *, *, #1237, .T. ) ;
#2616=ORIENTED_EDGE ( 'NONE', *, *, #2459, .T. ) ;
#2618=ORIENTED_EDGE ( 'NONE', *, *, #12520, .F. ) ;
#2626=CARTESIAN_POINT ( 'NONE',  ( -91.14322581977729953, 6.938893903907228378E-15, 6.823838874241844543 ) ) ;
#2627=DIRECTION ( 'NONE',  ( -1.000000000000000000, -2.220446049250301001E-16, 0.000000000000000000 ) ) ;
#2629=CARTESIAN_POINT ( 'NONE',  ( -50.65685424949267457, 7.200000000000018829, -7.500000000000034639 ) ) ;
#2636=DIRECTION ( 'NONE',  ( 1.000000000000000000, 2.168404344970992105E-16, -5.204170427930381051E-15 ) ) ;
#2642=VECTOR ( 'NONE', #1442, 1000.000000000000000 ) ;
#2646=ORIENTED_EDGE ( 'NONE', *, *, #3704, .F. ) ;
#2649=LINE ( 'NONE', #16753, #21587 ) ;
#2650=ADVANCED_FACE ( 'NONE', ( #4411 ), #21010, .T. ) ;
#2652=VERTEX_POINT ( 'NONE', #15466 ) ;
#2657=CARTESIAN_POINT ( 'NONE',  ( -47.82842712474658242, 4.371572875253824542, -7.500000000000007105 ) ) ;
#2661=FACE_BOUND ( 'NONE', #20938, .T. ) ;
#2663=EDGE_CURVE ( 'NONE', #9669, #7684, #12697, .T. ) ;
#2671=ORIENTED_EDGE ( 'NONE', *, *, #17854, .T. ) ;
#2672=ORIENTED_EDGE ( 'NONE', *, *, #557, .T. ) ;
#2674=CARTESIAN_POINT ( 'NONE',  ( -42.54314575050782565, -7.500000000000038192, -8.000000000000007105 ) ) ;
#2680=DIRECTION ( 'NONE',  ( -2.013525853228507892E-32, -6.902532920683810383E-31, 1.000000000000000000 ) ) ;
#2686=CIRCLE ( 'NONE', #3811, 0.5000000000000028866 ) ;
#2689=LINE ( 'NONE', #20583, #5218 ) ;
#2690=DIRECTION ( 'NONE',  ( -1.000000000000000000, 1.387778780781435420E-14, 9.144641450333394555E-31 ) ) ;
#2703=FACE_OUTER_BOUND ( 'NONE', #18173, .T. ) ;
#2704=DIRECTION ( 'NONE',  ( -0.6666666666666649643, -2.585973076299232148E-15, -0.7453559924999314523 ) ) ;
#2709=LINE ( 'NONE', #4826, #17444 ) ;
#2711=DIRECTION ( 'NONE',  ( 2.013525853228508439E-32, 6.779273404243028164E-31, -1.000000000000000000 ) ) ;
#2716=CIRCLE ( 'NONE', #19635, 2.500000000000015987 ) ;
#2727=AXIS2_PLACEMENT_3D ( 'NONE', #13546, #2957, #12109 ) ;
#2736=AXIS2_PLACEMENT_3D ( 'NONE', #13824, #10172, #12398 ) ;
#2748=DIRECTION ( 'NONE',  ( 2.013525853228507892E-32, 6.902532920683810383E-31, -1.000000000000000000 ) ) ;
#2754=VECTOR ( 'NONE', #7282, 1000.000000000000114 ) ;
#2762=ORIENTED_EDGE ( 'NONE', *, *, #1632, .T. ) ;
#2764=ORIENTED_EDGE ( 'NONE', *, *, #13415, .T. ) ;
#2772=DIRECTION ( 'NONE',  ( 2.013525853228507892E-32, 6.902532920683810383E-31, -1.000000000000000000 ) ) ;
#2803=EDGE_CURVE ( 'NONE', #18939, #11087, #17601, .T. ) ;
#2809=CARTESIAN_POINT ( 'NONE',  ( -89.70000000000065654, 3.200000000000057021, -2.000000000000001776 ) ) ;
#2811=DIRECTION ( 'NONE',  ( 1.550910762415566494E-16, 1.000000000000000000, -8.135128085091684243E-31 ) ) ;
#2819=FACE_OUTER_BOUND ( 'NONE', #1943, .T. ) ;
#2824=VECTOR ( 'NONE', #8683, 1000.000000000000000 ) ;
#2827=AXIS2_PLACEMENT_3D ( 'NONE', #4818, #19172, #20946 ) ;
#2832=VERTEX_POINT ( 'NONE', #17696 ) ;
#2834=CARTESIAN_POINT ( 'NONE',  ( -42.54314575050793934, 7.999999999999992895, -7.500000000000062172 ) ) ;
#2840=LINE ( 'NONE', #3198, #19094 ) ;
#2842=DIRECTION ( 'NONE',  ( -1.000000000000000000, 1.626303258728243832E-16, -4.409088834774349725E-15 ) ) ;
#2848=VERTEX_POINT ( 'NONE', #5119 ) ;
#2860=CARTESIAN_POINT ( 'NONE',  ( -95.20000000000058549, -2.700000000000119194, 8.000000000000035527 ) ) ;
#2861=AXIS2_PLACEMENT_3D ( 'NONE', #21866, #5758, #13040 ) ;
#2863=FACE_OUTER_BOUND ( 'NONE', #10572, .T. ) ;
#2869=CARTESIAN_POINT ( 'NONE',  ( -65.00000000000052580, 0.5000000000000490719, 3.000000000000002665 ) ) ;
#2873=ORIENTED_EDGE ( 'NONE', *, *, #15785, .T. ) ;
#2878=EDGE_LOOP ( 'NONE', ( #691, #4951, #9968, #17787 ) ) ;
#2890=DIRECTION ( 'NONE',  ( 2.013525853228508439E-32, 6.779273404243028164E-31, -1.000000000000000000 ) ) ;
#2893=CARTESIAN_POINT ( 'NONE',  ( -50.65685424949267457, 7.200000000000018829, -7.500000000000034639 ) ) ;
#2902=CARTESIAN_POINT ( 'NONE',  ( -50.65685424949267457, -7.200000000000049916, 7.500000000000047962 ) ) ;
#2906=AXIS2_PLACEMENT_3D ( 'NONE', #768, #2748, #15089 ) ;
#2913=VERTEX_POINT ( 'NONE', #5248 ) ;
#2914=CIRCLE ( 'NONE', #7798, 0.5000000000000004441 ) ;
#2915=DIRECTION ( 'NONE',  ( 0.000000000000000000, -1.000000000000000000, 0.000000000000000000 ) ) ;
#2916=CARTESIAN_POINT ( 'NONE',  ( -53.99613665484953628, -0.5000000000001045830, -13.19342998475053719 ) ) ;
#2917=TOROIDAL_SURFACE ( 'NONE', #23220, 5.500000000000007994, 0.5000000000000000000 ) ;
#2920=EDGE_CURVE ( 'NONE', #12385, #6815, #20246, .T. ) ;
#2923=AXIS2_PLACEMENT_3D ( 'NONE', #20338, #20108, #21872 ) ;
#2931=CARTESIAN_POINT ( 'NONE',  ( -95.20000000000064233, 3.200000000000015277, 1.000000000000014655 ) ) ;
#2935=CIRCLE ( 'NONE', #23236, 5.500000000000032863 ) ;
#2936=ORIENTED_EDGE ( 'NONE', *, *, #2964, .T. ) ;
#2943=AXIS2_PLACEMENT_3D ( 'NONE', #4719, #11775, #10135 ) ;
#2944=ORIENTED_EDGE ( 'NONE', *, *, #12592, .F. ) ;
#2945=ORIENTED_EDGE ( 'NONE', *, *, #22642, .F. ) ;
#2946=CIRCLE ( 'NONE', #8960, 0.5000000000000004441 ) ;
#2948=DIRECTION ( 'NONE',  ( -1.110223024625150131E-16, 1.000000000000000000, -6.902532920683853297E-31 ) ) ;
#2949=DIRECTION ( 'NONE',  ( 2.013525853228507892E-32, 6.902532920683810383E-31, -1.000000000000000000 ) ) ;
#2957=DIRECTION ( 'NONE',  ( 0.7071067811865485719, -0.7071067811865464625, -1.010793663541191362E-16 ) ) ;
#2961=DIRECTION ( 'NONE',  ( -1.000000000000000000, 1.550910762415513985E-16, 3.012982189080959477E-32 ) ) ;
#2963=DIRECTION ( 'NONE',  ( 0.000000000000000000, 0.000000000000000000, 1.000000000000000000 ) ) ;
#2964=EDGE_CURVE ( 'NONE', #8098, #21208, #18288, .T. ) ;
#2969=ORIENTED_EDGE ( 'NONE', *, *, #6054, .T. ) ;
#2976=DIRECTION ( 'NONE',  ( -1.000000000000000000, 1.550910762415516450E-16, 0.000000000000000000 ) ) ;
#2980=CARTESIAN_POINT ( 'NONE',  ( -55.25320565519145788, -2.700000000000049472, 8.000000000000062172 ) ) ;
#2982=DIRECTION ( 'NONE',  ( 0.7071067811865491270, 0.7071067811865461294, 1.565905175853767167E-16 ) ) ;
#2989=CARTESIAN_POINT ( 'NONE',  ( -42.54314575050793934, 7.999999999999992895, -7.500000000000062172 ) ) ;
#2994=ORIENTED_EDGE ( 'NONE', *, *, #15001, .T. ) ;
#3000=VERTEX_POINT ( 'NONE', #16276 ) ;
#3001=ORIENTED_EDGE ( 'NONE', *, *, #16818, .F. ) ;
#3004=VERTEX_POINT ( 'NONE', #13218 ) ;
#3016=TOROIDAL_SURFACE ( 'NONE', #9030, 9.499999999999998224, 0.5000000000000000000 ) ;
#3023=ORIENTED_EDGE ( 'NONE', *, *, #23047, .F. ) ;
#3024=ADVANCED_FACE ( 'NONE', ( #189 ), #16504, .T. ) ;
#3029=ORIENTED_EDGE ( 'NONE', *, *, #474, .F. ) ;
#3034=AXIS2_PLACEMENT_3D ( 'NONE', #2629, #9804, #20638 ) ;
#3052=ADVANCED_FACE ( 'NONE', ( #10872 ), #18065, .T. ) ;
#3055=ADVANCED_FACE ( 'NONE', ( #2863 ), #11908, .T. ) ;
#3057=ORIENTED_EDGE ( 'NONE', *, *, #22635, .T. ) ;
#3058=DIRECTION ( 'NONE',  ( 2.013525853228507892E-32, 6.902532920683810383E-31, -1.000000000000000000 ) ) ;
#3071=DIRECTION ( 'NONE',  ( 1.550910762415566494E-16, 1.000000000000000000, -8.135128085091684243E-31 ) ) ;
#3082=AXIS2_PLACEMENT_3D ( 'NONE', #2448, #16902, #4440 ) ;
#3086=ORIENTED_EDGE ( 'NONE', *, *, #18849, .T. ) ;
#3095=MECHANICAL_DESIGN_GEOMETRIC_PRESENTATION_REPRESENTATION('',(#19997),#4958);
#3106=CYLINDRICAL_SURFACE ( 'NONE', #12675, 0.5000000000000038858 ) ;
#3110=EDGE_LOOP ( 'NONE', ( #13809, #15979, #12595, #2764 ) ) ;
#3120=CIRCLE ( 'NONE', #2368, 0.5000000000000004441 ) ;
#3121=CIRCLE ( 'NONE', #8370, 0.5000000000000028866 ) ;
#3122=TOROIDAL_SURFACE ( 'NONE', #121, 5.500000000000000000, 0.5000000000000000000 ) ;
#3125=CARTESIAN_POINT ( 'NONE',  ( -3.200000000000091660, -2.000000000000050182, -7.500000000000034639 ) ) ;
#3134=EDGE_CURVE ( 'NONE', #6825, #1880, #5299, .T. ) ;
#3136=DIRECTION ( 'NONE',  ( 1.000000000000000000, 2.220446049250314067E-16, -5.825996348268307008E-33 ) ) ;
#3137=CIRCLE ( 'NONE', #885, 2.500000000000015987 ) ;
#3138=VECTOR ( 'NONE', #18, 1000.000000000000000 ) ;
#3153=ORIENTED_EDGE ( 'NONE', *, *, #15877, .F. ) ;
#3156=TOROIDAL_SURFACE ( 'NONE', #9161, 3.299999999999999822, 0.5000000000000000000 ) ;
#3162=AXIS2_PLACEMENT_3D ( 'NONE', #576, #7741, #18336 ) ;
#3165=DIRECTION ( 'NONE',  ( -2.013525853228507892E-32, -6.902532920683810383E-31, 1.000000000000000000 ) ) ;
#3168=CARTESIAN_POINT ( 'NONE',  ( -42.54314575050785407, -5.300000000000020250, 8.000000000000007105 ) ) ;
#3171=EDGE_CURVE ( 'NONE', #17679, #9575, #19992, .T. ) ;
#3174=VECTOR ( 'NONE', #17205, 1000.000000000000000 ) ;
#3183=CARTESIAN_POINT ( 'NONE',  ( -47.47487373415315659, -4.018019484660608320, -8.000000000000007105 ) ) ;
#3186=CARTESIAN_POINT ( 'NONE',  ( -64.00000000000045475, 3.200000000000057021, -1.999999999999974021 ) ) ;
#3197=DIRECTION ( 'NONE',  ( 2.710505431213761578E-16, -1.000000000000000000, 7.518830502887770522E-31 ) ) ;
#3198=CARTESIAN_POINT ( 'NONE',  ( -3.200000000000133404, 1.999999999999953149, -8.000000000000035527 ) ) ;
#3199=CARTESIAN_POINT ( 'NONE',  ( -47.82842712474649716, 4.371572875253824542, 8.000000000000021316 ) ) ;
#3200=ADVANCED_FACE ( 'NONE', ( #7078 ), #14474, .F. ) ;
#3207=ADVANCED_FACE ( 'NONE', ( #7307 ), #14583, .F. ) ;
#3212=VERTEX_POINT ( 'NONE', #5882 ) ;
#3213=DIRECTION ( 'NONE',  ( 1.331202777560457422E-30, 1.000000000000000000, -7.395570986446985676E-31 ) ) ;
#3221=EDGE_CURVE ( 'NONE', #10966, #5384, #3668, .T. ) ;
#3226=FACE_OUTER_BOUND ( 'NONE', #22419, .T. ) ;
#3228=DIRECTION ( 'NONE',  ( -1.000000000000000000, -1.479114197289388027E-30, 2.013525853228518840E-32 ) ) ;
#3229=CARTESIAN_POINT ( 'NONE',  ( -42.54314575050793934, 7.499999999999992895, 8.000000000000035527 ) ) ;
#3240=ORIENTED_EDGE ( 'NONE', *, *, #9671, .T. ) ;
#3245=PLANE ( 'NONE',  #6123 ) ;
#3248=LINE ( 'NONE', #1250, #17370 ) ;
#3261=CIRCLE ( 'NONE', #5128, 0.5000000000000029976 ) ;
#3269=ORIENTED_EDGE ( 'NONE', *, *, #1818, .F. ) ;
#3273=LINE ( 'NONE', #14084, #6860 ) ;
#3277=LINE ( 'NONE', #1729, #17593 ) ;
#3279=FACE_OUTER_BOUND ( 'NONE', #6126, .T. ) ;
#3282=CARTESIAN_POINT ( 'NONE',  ( -3.200000000000091660, -2.000000000000043521, 7.500000000000047962 ) ) ;
#3285=LINE ( 'NONE', #4514, #2201 ) ;
#3302=DIRECTION ( 'NONE',  ( -2.220446049250313081E-16, 1.000000000000000000, -7.025792437124636392E-31 ) ) ;
#3304=ORIENTED_EDGE ( 'NONE', *, *, #8695, .T. ) ;
#3308=AXIS2_PLACEMENT_3D ( 'NONE', #22985, #3449, #14273 ) ;
#3322=CIRCLE ( 'NONE', #10815, 0.5000000000000029976 ) ;
#3328=EDGE_CURVE ( 'NONE', #21722, #16175, #10051, .T. ) ;
#3330=DIRECTION ( 'NONE',  ( -1.000000000000000000, 1.550910762415566494E-16, -8.566929763922626680E-48 ) ) ;
#3331=DIRECTION ( 'NONE',  ( -0.7071067811865490160, -0.7071067811865460184, -1.565905175853766674E-16 ) ) ;
#3333=CARTESIAN_POINT ( 'NONE',  ( -6.000000000000130562, 5.299999999999957190, -8.000000000000035527 ) ) ;
#3337=FACE_OUTER_BOUND ( 'NONE', #22877, .T. ) ;
#3339=CARTESIAN_POINT ( 'NONE',  ( -42.54314575050793934, -4.000000000000021316, 7.500000000000062172 ) ) ;
#3341=VECTOR ( 'NONE', #7356, 1000.000000000000000 ) ;
#3345=EDGE_CURVE ( 'NONE', #13984, #18025, #2914, .T. ) ;
#3354=ORIENTED_EDGE ( 'NONE', *, *, #20656, .T. ) ;
#3361=EDGE_LOOP ( 'NONE', ( #11658, #10861, #15972, #630 ) ) ;
#3362=ORIENTED_EDGE ( 'NONE', *, *, #15001, .F. ) ;
#3365=ORIENTED_EDGE ( 'NONE', *, *, #11287, .T. ) ;
#3366=CARTESIAN_POINT ( 'NONE',  ( -55.25320565519145788, 9.020562075079396891E-14, 10.00000000000009237 ) ) ;
#3375=EDGE_CURVE ( 'NONE', #9172, #5639, #16048, .T. ) ;
#3376=AXIS2_PLACEMENT_3D ( 'NONE', #14373, #3673, #1682 ) ;
#3392=EDGE_CURVE ( 'NONE', #22415, #9172, #17263, .T. ) ;
#3395=CARTESIAN_POINT ( 'NONE',  ( -50.65685424949267457, -7.200000000000049916, 8.000000000000035527 ) ) ;
#3407=CIRCLE ( 'NONE', #6412, 2.550000000000010481 ) ;
#3414=DIRECTION ( 'NONE',  ( 1.000000000000000000, 2.168404344970992105E-16, 0.000000000000000000 ) ) ;
#3415=DIRECTION ( 'NONE',  ( -2.220446049250313081E-16, 1.000000000000000000, -7.025792437124636392E-31 ) ) ;
#3416=DIRECTION ( 'NONE',  ( 0.7071067811865485719, -0.7071067811865464625, -1.010793663541191485E-16 ) ) ;
#3418=CARTESIAN_POINT ( 'NONE',  ( -45.56568542494949980, 0.5000000000000559552, -7.500000000000007105 ) ) ;
#3423=LINE ( 'NONE', #20, #10327 ) ;
#3433=ORIENTED_EDGE ( 'NONE', *, *, #3838, .F. ) ;
#3436=AXIS2_PLACEMENT_3D ( 'NONE', #15590, #19235, #17590 ) ;
#3439=LINE ( 'NONE', #454, #22988 ) ;
#3445=DIRECTION ( 'NONE',  ( -1.000000000000000000, 1.409462824231139829E-14, 0.000000000000000000 ) ) ;
#3449=DIRECTION ( 'NONE',  ( 1.000000000000000000, 1.479114197289388027E-30, -2.013525853228518840E-32 ) ) ;
#3455=EDGE_CURVE ( 'NONE', #21891, #15244, #13752, .T. ) ;
#3458=ORIENTED_EDGE ( 'NONE', *, *, #20035, .T. ) ;
#3466=VECTOR ( 'NONE', #22189, 1000.000000000000000 ) ;
#3469=CIRCLE ( 'NONE', #11737, 6.000000000000047073 ) ;
#3477=TOROIDAL_SURFACE ( 'NONE', #18118, 9.499999999999998224, 0.5000000000000000000 ) ;
#3479=FACE_OUTER_BOUND ( 'NONE', #7877, .T. ) ;
#3480=VERTEX_POINT ( 'NONE', #3282 ) ;
#3493=EDGE_LOOP ( 'NONE', ( #8371, #1521, #6300, #20864 ) ) ;
#3495=FACE_OUTER_BOUND ( 'NONE', #12885, .T. ) ;
#3498=VECTOR ( 'NONE', #14349, 1000.000000000000000 ) ;
#3499=CARTESIAN_POINT ( 'NONE',  ( -42.54314575050793934, 4.799999999999998934, 7.500000000000062172 ) ) ;
#3507=EDGE_CURVE ( 'NONE', #5668, #11952, #11551, .T. ) ;
#3509=EDGE_CURVE ( 'NONE', #18638, #9788, #19382, .T. ) ;
#3513=CARTESIAN_POINT ( 'NONE',  ( -6.000000000000116351, -8.000000000000003553, -8.000000000000007105 ) ) ;
#3519=AXIS2_PLACEMENT_3D ( 'NONE', #3751, #240, #2103 ) ;
#3522=AXIS2_PLACEMENT_3D ( 'NONE', #18916, #17130, #22443 ) ;
#3526=EDGE_LOOP ( 'NONE', ( #9450, #17571, #30, #2037 ) ) ;
#3528=EDGE_CURVE ( 'NONE', #2913, #5438, #20588, .T. ) ;
#3534=ORIENTED_EDGE ( 'NONE', *, *, #817, .F. ) ;
#3545=CARTESIAN_POINT ( 'NONE',  ( -6.000000000000019540, -5.300000000000006040, 7.500000000000062172 ) ) ;
#3550=ORIENTED_EDGE ( 'NONE', *, *, #472, .T. ) ;
#3551=EDGE_CURVE ( 'NONE', #22821, #1743, #14561, .T. ) ;
#3565=CARTESIAN_POINT ( 'NONE',  ( -55.25320565519140104, -2.700000000000049472, 10.00000000000007816 ) ) ;
#3573=DIRECTION ( 'NONE',  ( 1.000000000000000000, 2.168404344970995063E-16, 0.000000000000000000 ) ) ;
#3575=ORIENTED_EDGE ( 'NONE', *, *, #7959, .F. ) ;
#3579=VERTEX_POINT ( 'NONE', #8918 ) ;
#3588=AXIS2_PLACEMENT_3D ( 'NONE', #9889, #6128, #13305 ) ;
#3590=DIRECTION ( 'NONE',  ( -1.000000000000000000, 0.000000000000000000, 0.000000000000000000 ) ) ;
#3592=EDGE_CURVE ( 'NONE', #17679, #14402, #9311, .T. ) ;
#3595=CARTESIAN_POINT ( 'NONE',  ( -6.000000000000143885, -2.000000000000043521, 8.000000000000062172 ) ) ;
#3599=CARTESIAN_POINT ( 'NONE',  ( -50.65685424949274562, -2.700000000000125855, 7.500000000000076383 ) ) ;
#3601=FACE_OUTER_BOUND ( 'NONE', #15852, .T. ) ;
#3625=EDGE_CURVE ( 'NONE', #21208, #9368, #2935, .T. ) ;
#3630=AXIS2_PLACEMENT_3D ( 'NONE', #21717, #9123, #16284 ) ;
#3647=CARTESIAN_POINT ( 'NONE',  ( -6.000000000000143885, -2.000000000000043521, 8.000000000000062172 ) ) ;
#3648=CARTESIAN_POINT ( 'NONE',  ( -43.10883117545713361, -5.300000000000020250, 8.000000000000035527 ) ) ;
#3649=DIRECTION ( 'NONE',  ( -1.000000000000000000, 1.550910762415521134E-16, -6.938893903907184004E-16 ) ) ;
#3653=ADVANCED_FACE ( 'NONE', ( #14666 ), #12306, .T. ) ;
#3655=EDGE_LOOP ( 'NONE', ( #11959, #302 ) ) ;
#3660=EDGE_LOOP ( 'NONE', ( #2390, #3354, #5229, #4788 ) ) ;
#3661=CIRCLE ( 'NONE', #22437, 0.5000000000000028866 ) ;
#3664=CARTESIAN_POINT ( 'NONE',  ( -42.54314575050793934, 7.499999999999992895, -7.500000000000062172 ) ) ;
#3667=DIRECTION ( 'NONE',  ( 0.7071067811865457964, -0.7071067811865492381, 0.000000000000000000 ) ) ;
#3668=CIRCLE ( 'NONE', #22445, 0.8000000000000090372 ) ;
#3673=DIRECTION ( 'NONE',  ( 1.000000000000000000, 1.133987551255197989E-30, 1.404432126150814977E-14 ) ) ;
#3675=PLANE ( 'NONE',  #890 ) ;
#3681=DIRECTION ( 'NONE',  ( 1.144237745221811361E-17, -1.000000000000000000, 7.025792437124636392E-31 ) ) ;
#3704=EDGE_CURVE ( 'NONE', #11087, #20601, #20438, .T. ) ;
#3705=DIRECTION ( 'NONE',  ( -6.938893903907264665E-15, 1.000000000000000000, 7.642090019328551865E-31 ) ) ;
#3707=CARTESIAN_POINT ( 'NONE',  ( -3.200000000000133404, -2.000000000000008882, -8.000000000000035527 ) ) ;
#3714=ORIENTED_EDGE ( 'NONE', *, *, #8110, .F. ) ;
#3715=ADVANCED_FACE ( 'NONE', ( #22319 ), #13372, .F. ) ;
#3718=LINE ( 'NONE', #5852, #11031 ) ;
#3719=CARTESIAN_POINT ( 'NONE',  ( -6.000000000000088818, -2.000000000000050182, -17.72029585817572084 ) ) ;
#3720=CARTESIAN_POINT ( 'NONE',  ( -42.54314575050782565, -4.800000000000037126, -8.000000000000007105 ) ) ;
#3726=CARTESIAN_POINT ( 'NONE',  ( -67.40537636629476026, -2.700000000000125855, 12.70639812373640432 ) ) ;
#3727=DIRECTION ( 'NONE',  ( -1.550910762415566494E-16, -1.000000000000000000, 8.135128085091684243E-31 ) ) ;
#3736=ORIENTED_EDGE ( 'NONE', *, *, #9240, .T. ) ;
#3743=LINE ( 'NONE', #15855, #4704 ) ;
#3751=CARTESIAN_POINT ( 'NONE',  ( -6.000000000000088818, -2.000000000000043521, -7.500000000000007105 ) ) ;
#3757=EDGE_CURVE ( 'NONE', #13088, #2421, #11135, .T. ) ;
#3758=DIRECTION ( 'NONE',  ( -1.000000000000000000, 1.734723475976796001E-16, 0.000000000000000000 ) ) ;
#3764=ORIENTED_EDGE ( 'NONE', *, *, #16718, .T. ) ;
#3765=ORIENTED_EDGE ( 'NONE', *, *, #12267, .T. ) ;
#3768=ADVANCED_FACE ( 'NONE', ( #14897 ), #5975, .T. ) ;
#3782=ADVANCED_FACE ( 'NONE', ( #8074, #2661, #6554 ), #18900, .F. ) ;
#3797=EDGE_LOOP ( 'NONE', ( #17358, #22679, #6385, #5162 ) ) ;
#3799=ADVANCED_FACE ( 'NONE', ( #15232 ), #17348, .T. ) ;
#3800=EDGE_LOOP ( 'NONE', ( #10927, #16895, #13953, #20041 ) ) ;
#3808=CARTESIAN_POINT ( 'NONE',  ( -42.54314575050799618, 7.499999999999992895, 8.000000000000035527 ) ) ;
#3811=AXIS2_PLACEMENT_3D ( 'NONE', #14894, #4178, #20205 ) ;
#3820=ORIENTED_EDGE ( 'NONE', *, *, #18929, .T. ) ;
#3821=ORIENTED_EDGE ( 'NONE', *, *, #3936, .T. ) ;
#3825=ORIENTED_EDGE ( 'NONE', *, *, #9739, .T. ) ;
#3826=ORIENTED_EDGE ( 'NONE', *, *, #6550, .F. ) ;
#3838=EDGE_CURVE ( 'NONE', #1775, #19103, #22548, .T. ) ;
#3841=CYLINDRICAL_SURFACE ( 'NONE', #2906, 0.5000000000000004441 ) ;
#3845=CIRCLE ( 'NONE', #19262, 0.5000000000000038858 ) ;
#3846=CARTESIAN_POINT ( 'NONE',  ( -42.54314575050796776, 3.999999999999996447, -8.000000000000035527 ) ) ;
#3850=CARTESIAN_POINT ( 'NONE',  ( -89.70000000000054285, -6.245004513516505540E-14, 1.000000000000000888 ) ) ;
#3854=DIRECTION ( 'NONE',  ( -2.013525853228507892E-32, -6.902532920683810383E-31, 1.000000000000000000 ) ) ;
#3866=EDGE_CURVE ( 'NONE', #9788, #4065, #12350, .T. ) ;
#3873=FACE_OUTER_BOUND ( 'NONE', #10394, .T. ) ;
#3876=AXIS2_PLACEMENT_3D ( 'NONE', #873, #8043, #22397 ) ;
#3886=LINE ( 'NONE', #18473, #22378 ) ;
#3890=DIRECTION ( 'NONE',  ( -0.7071067811865507924, -0.7071067811865444641, 7.226392596171890537E-15 ) ) ;
#3891=TOROIDAL_SURFACE ( 'NONE', #8033, 6.700000000000001066, 0.5000000000000000000 ) ;
#3893=VECTOR ( 'NONE', #19141, 1000.000000000000000 ) ;
#3894=CARTESIAN_POINT ( 'NONE',  ( -56.87767137932630845, -0.5000000000000281997, 8.833333333333401427 ) ) ;
#3896=DIRECTION ( 'NONE',  ( 0.000000000000000000, 1.000000000000000000, 0.000000000000000000 ) ) ;
#3900=LINE ( 'NONE', #20498, #4673 ) ;
#3921=ORIENTED_EDGE ( 'NONE', *, *, #23210, .F. ) ;
#3925=DIRECTION ( 'NONE',  ( 1.000000000000000000, -1.550910762415513985E-16, -3.012982189080959477E-32 ) ) ;
#3926=LINE ( 'NONE', #3808, #9397 ) ;
#3928=AXIS2_PLACEMENT_3D ( 'NONE', #1194, #4936, #10013 ) ;
#3935=CARTESIAN_POINT ( 'NONE',  ( -45.56568542494964191, 2.108831175456925333, -8.000000000000062172 ) ) ;
#3936=EDGE_CURVE ( 'NONE', #1743, #10125, #8235, .T. ) ;
#3938=EDGE_CURVE ( 'NONE', #23066, #9452, #17236, .T. ) ;
#3939=ORIENTED_EDGE ( 'NONE', *, *, #6350, .T. ) ;
#3946=ORIENTED_EDGE ( 'NONE', *, *, #20317, .F. ) ;
#3951=DIRECTION ( 'NONE',  ( -1.331202777560457422E-30, -1.000000000000000000, 7.395570986446985676E-31 ) ) ;
#3953=DIRECTION ( 'NONE',  ( -1.000000000000000000, 1.550910762415526064E-16, 0.000000000000000000 ) ) ;
#3954=DIRECTION ( 'NONE',  ( -0.7071067811865457964, -0.7071067811865492381, 0.000000000000000000 ) ) ;
#3984=DIRECTION ( 'NONE',  ( 2.013525853228507892E-32, 6.902532920683810383E-31, -1.000000000000000000 ) ) ;
#3985=DIRECTION ( 'NONE',  ( -1.000000000000000000, 3.469446951953575061E-14, 0.000000000000000000 ) ) ;
#3986=DIRECTION ( 'NONE',  ( -1.000000000000000000, -1.479114197289387852E-30, 2.013525853228518840E-32 ) ) ;
#3992=AXIS2_PLACEMENT_3D ( 'NONE', #13338, #20637, #2505 ) ;
#3998=ORIENTED_EDGE ( 'NONE', *, *, #10158, .T. ) ;
#4007=CARTESIAN_POINT ( 'NONE',  ( -45.56568542494954244, -2.700000000000091216, -7.500000000000062172 ) ) ;
#4011=CARTESIAN_POINT ( 'NONE',  ( -43.10883117545713361, -4.565685424949276872, 8.000000000000035527 ) ) ;
#4015=AXIS2_PLACEMENT_3D ( 'NONE', #18838, #8023, #13436 ) ;
#4017=CARTESIAN_POINT ( 'NONE',  ( -50.65685424949281668, 1.387778780781445676E-14, 7.500000000000034639 ) ) ;
#4024=ORIENTED_EDGE ( 'NONE', *, *, #13838, .T. ) ;
#4027=ORIENTED_EDGE ( 'NONE', *, *, #15274, .T. ) ;
#4033=ORIENTED_EDGE ( 'NONE', *, *, #19604, .F. ) ;
#4035=LINE ( 'NONE', #14406, #173 ) ;
#4036=EDGE_CURVE ( 'NONE', #21802, #18939, #16057, .T. ) ;
#4039=CARTESIAN_POINT ( 'NONE',  ( -64.00000000000045475, -0.5000000000000628386, -2.000000000000001776 ) ) ;
#4040=EDGE_CURVE ( 'NONE', #16175, #15826, #19720, .T. ) ;
#4046=VECTOR ( 'NONE', #11331, 1000.000000000000114 ) ;
#4048=AXIS2_PLACEMENT_3D ( 'NONE', #9153, #21517, #23046 ) ;
#4063=CIRCLE ( 'NONE', #10083, 0.5000000000000000000 ) ;
#4065=VERTEX_POINT ( 'NONE', #16392 ) ;
#4071=DIRECTION ( 'NONE',  ( 1.000000000000000000, -1.389842848855773367E-62, 2.013525853228507892E-32 ) ) ;
#4084=FACE_OUTER_BOUND ( 'NONE', #4644, .T. ) ;
#4089=CYLINDRICAL_SURFACE ( 'NONE', #8335, 0.5000000000000004441 ) ;
#4092=CARTESIAN_POINT ( 'NONE',  ( -6.000000000000074607, -8.000000000000003553, -7.500000000000034639 ) ) ;
#4118=DIRECTION ( 'NONE',  ( -2.013525853228507892E-32, -6.902532920683810383E-31, 1.000000000000000000 ) ) ;
#4121=CARTESIAN_POINT ( 'NONE',  ( -55.25320565519152893, 2.700000000000104983, 8.000000000000035527 ) ) ;
#4131=DIRECTION ( 'NONE',  ( -0.7071067811865535679, -0.7071067811865414665, 0.000000000000000000 ) ) ;
#4138=ORIENTED_EDGE ( 'NONE', *, *, #4784, .F. ) ;
#4139=VERTEX_POINT ( 'NONE', #9466 ) ;
#4141=EDGE_LOOP ( 'NONE', ( #8555, #21837, #8518, #10796 ) ) ;
#4144=VERTEX_POINT ( 'NONE', #16857 ) ;
#4157=LINE ( 'NONE', #3935, #4046 ) ;
#4162=DIRECTION ( 'NONE',  ( 1.000000000000000000, 2.220446049250313081E-16, -3.656342123407104498E-48 ) ) ;
#4165=VERTEX_POINT ( 'NONE', #298 ) ;
#4167=EDGE_CURVE ( 'NONE', #7485, #21891, #4157, .T. ) ;
#4170=DIRECTION ( 'NONE',  ( 0.9878135252003127365, 2.193386639427060722E-16, -0.1556420233463029767 ) ) ;
#4178=DIRECTION ( 'NONE',  ( 0.9706398123736300620, 1.281898970984135951E-30, 0.2405376366294562085 ) ) ;
#4184=CARTESIAN_POINT ( 'NONE',  ( -50.65685424949263904, -7.200000000000071232, -7.500000000000034639 ) ) ;
#4203=DIRECTION ( 'NONE',  ( -1.000000000000000000, 1.550910762415566494E-16, 1.495339968488870838E-47 ) ) ;
#4211=EDGE_CURVE ( 'NONE', #23028, #278, #1418, .T. ) ;
#4220=CIRCLE ( 'NONE', #118, 0.5000000000000004441 ) ;
#4225=ORIENTED_EDGE ( 'NONE', *, *, #22624, .T. ) ;
#4226=CARTESIAN_POINT ( 'NONE',  ( -65.47859922179029013, -0.5000000000000628386, -11.38422848940298593 ) ) ;
#4229=FACE_OUTER_BOUND ( 'NONE', #1355, .T. ) ;
#4239=CIRCLE ( 'NONE', #139, 0.5000000000000029976 ) ;
#4255=AXIS2_PLACEMENT_3D ( 'NONE', #70, #16383, #7467 ) ;
#4258=ORIENTED_EDGE ( 'NONE', *, *, #11390, .T. ) ;
#4266=CARTESIAN_POINT ( 'NONE',  ( -45.37157287525408833, -6.828427124746183630, -7.500000000000034639 ) ) ;
#4281=VERTEX_POINT ( 'NONE', #20876 ) ;
#4290=CARTESIAN_POINT ( 'NONE',  ( -91.14322581977724269, -0.5000000000001045830, 6.823838874241872077 ) ) ;
#4291=VERTEX_POINT ( 'NONE', #2989 ) ;
#4293=FACE_OUTER_BOUND ( 'NONE', #14730, .T. ) ;
#4299=CARTESIAN_POINT ( 'NONE',  ( -2.700000000000091216, -6.938893903907228378E-14, 7.500000000000117240 ) ) ;
#4312=FACE_OUTER_BOUND ( 'NONE', #5724, .T. ) ;
#4318=EDGE_CURVE ( 'NONE', #19103, #1910, #17947, .T. ) ;
#4327=CARTESIAN_POINT ( 'NONE',  ( -87.15000000000057412, -9.060110299520994546E-14, -2.000000000000002220 ) ) ;
#4342=EDGE_CURVE ( 'NONE', #16028, #6492, #10434, .T. ) ;
#4349=DIRECTION ( 'NONE',  ( 1.000000000000000000, 1.479114197289388027E-30, -2.013525853228518840E-32 ) ) ;
#4353=CARTESIAN_POINT ( 'NONE',  ( -90.55603112840533697, 3.200000000000057021, -7.432974388601714999 ) ) ;
#4360=EDGE_CURVE ( 'NONE', #6874, #19780, #10615, .T. ) ;
#4361=ORIENTED_EDGE ( 'NONE', *, *, #10211, .F. ) ;
#4362=ORIENTED_EDGE ( 'NONE', *, *, #197, .F. ) ;
#4364=EDGE_LOOP ( 'NONE', ( #15796, #512, #16491, #17960 ) ) ;
#4366=VERTEX_POINT ( 'NONE', #6746 ) ;
#4367=ORIENTED_EDGE ( 'NONE', *, *, #13056, .F. ) ;
#4369=EDGE_CURVE ( 'NONE', #2097, #9299, #3322, .T. ) ;
#4382=DIRECTION ( 'NONE',  ( -1.000000000000000000, -1.479114197289388027E-30, 2.013525853228518840E-32 ) ) ;
#4383=AXIS2_PLACEMENT_3D ( 'NONE', #22868, #19919, #11074 ) ;
#4402=ORIENTED_EDGE ( 'NONE', *, *, #817, .T. ) ;
#4408=ADVANCED_FACE ( 'NONE', ( #13916 ), #21102, .F. ) ;
#4411=FACE_OUTER_BOUND ( 'NONE', #3110, .T. ) ;
#4419=CIRCLE ( 'NONE', #2923, 2.550000000000010481 ) ;
#4422=EDGE_CURVE ( 'NONE', #14933, #2848, #6268, .T. ) ;
#4432=VERTEX_POINT ( 'NONE', #21345 ) ;
#4433=COLOUR_RGB ( '', 0.40784314, 0.44705882, 0.49803922) ;
#4434=CARTESIAN_POINT ( 'NONE',  ( -90.55603112840530855, 0.5000000000000490719, -7.432974388601742533 ) ) ;
#4440=DIRECTION ( 'NONE',  ( -1.000000000000000000, 1.703746271048639119E-15, 0.000000000000000000 ) ) ;
#4442=DIRECTION ( 'NONE',  ( -2.220446049250313081E-16, 1.000000000000000000, -7.025792437124636392E-31 ) ) ;
#4444=DIRECTION ( 'NONE',  ( 0.9878135252003127365, -1.532010627492774434E-16, -0.1556420233463029767 ) ) ;
#4445=AXIS2_PLACEMENT_3D ( 'NONE', #12636, #10757, #6890 ) ;
#4451=DIRECTION ( 'NONE',  ( -0.7071067811865490160, -0.7071067811865460184, -1.565905175853766674E-16 ) ) ;
#4452=CARTESIAN_POINT ( 'NONE',  ( -65.47859922179024750, -2.700000000000091216, -11.38422848940306942 ) ) ;
#4453=DIRECTION ( 'NONE',  ( 1.000000000000000000, 2.168404344970991858E-16, -9.035018104045799943E-16 ) ) ;
#4456=ORIENTED_EDGE ( 'NONE', *, *, #12037, .F. ) ;
#4470=DIRECTION ( 'NONE',  ( 1.387778780781445676E-14, -1.000000000000000000, 0.000000000000000000 ) ) ;
#4471=DIRECTION ( 'NONE',  ( -1.000000000000000000, -1.479114197289387852E-30, 2.013525853228518840E-32 ) ) ;
#4480=CARTESIAN_POINT ( 'NONE',  ( -65.00000000000052580, 3.200000000000057021, 3.000000000000002665 ) ) ;
#4485=PRODUCT_DEFINITION_FORMATION_WITH_SPECIFIED_SOURCE ( 'ANY', '', #13808, .NOT_KNOWN. ) ;
#4487=ADVANCED_FACE ( 'NONE', ( #17921 ), #15668, .F. ) ;
#4489=EDGE_LOOP ( 'NONE', ( #2579, #1152, #8344, #18053 ) ) ;
#4500=LINE ( 'NONE', #3720, #20165 ) ;
#4514=CARTESIAN_POINT ( 'NONE',  ( -45.37157287525418781, 6.828427124746204058, -8.000000000000035527 ) ) ;
#4519=ADVANCED_FACE ( 'NONE', ( #9323 ), #12845, .T. ) ;
#4526=EDGE_LOOP ( 'NONE', ( #8030, #16492, #3764, #6612 ) ) ;
#4528=LINE ( 'NONE', #16875, #1259 ) ;
#4533=DIRECTION ( 'NONE',  ( -1.000000000000000000, -1.479114197289388027E-30, 2.013525853228518840E-32 ) ) ;
#4541=ADVANCED_FACE ( 'NONE', ( #7558 ), #16364, .F. ) ;
#4549=AXIS2_PLACEMENT_3D ( 'NONE', #20339, #2811, #4203 ) ;
#4552=PLANE ( 'NONE',  #9871 ) ;
#4554=ORIENTED_EDGE ( 'NONE', *, *, #20162, .T. ) ;
#4559=CARTESIAN_POINT ( 'NONE',  ( -6.000000000000102141, 4.799999999999964295, 8.000000000000047962 ) ) ;
#4570=ORIENTED_EDGE ( 'NONE', *, *, #12459, .T. ) ;
#4572=AXIS2_PLACEMENT_3D ( 'NONE', #4011, #2019, #7669 ) ;
#4575=VECTOR ( 'NONE', #10673, 1000.000000000000000 ) ;
#4576=DIRECTION ( 'NONE',  ( -1.000000000000000000, 1.550910762415513985E-16, 3.012982189080959477E-32 ) ) ;
#4577=ADVANCED_FACE ( 'NONE', ( #7674 ), #1396, .T. ) ;
#4580=DIRECTION ( 'NONE',  ( 1.110223024625150131E-16, -1.000000000000000000, 6.902532920683853297E-31 ) ) ;
#4583=CARTESIAN_POINT ( 'NONE',  ( -56.91911807125098477, -2.700000000000084110, -8.333333333333413862 ) ) ;
#4596=CIRCLE ( 'NONE', #9884, 4.000000000000023981 ) ;
#4598=AXIS2_PLACEMENT_3D ( 'NONE', #3850, #1970, #5637 ) ;
#4603=VERTEX_POINT ( 'NONE', #4121 ) ;
#4604=ADVANCED_FACE ( 'NONE', ( #259 ), #20018, .T. ) ;
#4610=ADVANCED_FACE ( 'NONE', ( #4229 ), #18479, .T. ) ;
#4611=AXIS2_PLACEMENT_3D ( 'NONE', #18710, #11642, #2592 ) ;
#4635=EDGE_LOOP ( 'NONE', ( #10093, #2618, #1596, #22505 ) ) ;
#4637=AXIS2_PLACEMENT_3D ( 'NONE', #20982, #8859, #21457 ) ;
#4643=ORIENTED_EDGE ( 'NONE', *, *, #184, .F. ) ;
#4644=EDGE_LOOP ( 'NONE', ( #16117, #8849, #1006, #19831 ) ) ;
#4650=DIRECTION ( 'NONE',  ( -2.013525853228507892E-32, -6.902532920683810383E-31, 1.000000000000000000 ) ) ;
#4656=CARTESIAN_POINT ( 'NONE',  ( -2.700000000000091216, 1.999999999999946265, -7.500000000000034639 ) ) ;
#4662=DIRECTION ( 'NONE',  ( 2.655250634480531216E-32, -6.902532920683810383E-31, 1.000000000000000000 ) ) ;
#4664=DIRECTION ( 'NONE',  ( 2.013525853228507892E-32, 6.902532920683810383E-31, -1.000000000000000000 ) ) ;
#4670=AXIS2_PLACEMENT_3D ( 'NONE', #8858, #6990, #5325 ) ;
#4673=VECTOR ( 'NONE', #13194, 1000.000000000000000 ) ;
#4674=EDGE_LOOP ( 'NONE', ( #5669, #11410, #16266, #19571 ) ) ;
#4675=ORIENTED_EDGE ( 'NONE', *, *, #13532, .F. ) ;
#4676=AXIS2_PLACEMENT_3D ( 'NONE', #16270, #12629, #16497 ) ;
#4677=ORIENTED_EDGE ( 'NONE', *, *, #6379, .T. ) ;
#4678=CARTESIAN_POINT ( 'NONE',  ( -3.414274948570356294, 0.5000000000000628386, -21.66938530120590656 ) ) ;
#4681=DIRECTION ( 'NONE',  ( -1.000000000000000000, 1.424116703980815236E-16, 2.931272055834072749E-32 ) ) ;
#4691=CIRCLE ( 'NONE', #15943, 0.5000000000000028866 ) ;
#4692=CARTESIAN_POINT ( 'NONE',  ( -47.47487373415315659, -4.018019484660608320, -8.000000000000007105 ) ) ;
#4693=CIRCLE ( 'NONE', #11447, 6.700000000000039257 ) ;
#4694=DIRECTION ( 'NONE',  ( -1.000000000000000000, 1.734723475976796001E-16, 0.000000000000000000 ) ) ;
#4696=DIRECTION ( 'NONE',  ( 1.000000000000000000, 3.915518702919051914E-14, 0.000000000000000000 ) ) ;
#4704=VECTOR ( 'NONE', #14338, 1000.000000000000000 ) ;
#4717=DIRECTION ( 'NONE',  ( 1.000000000000000000, 2.775557561562873996E-14, 1.768522514469825155E-30 ) ) ;
#4719=CARTESIAN_POINT ( 'NONE',  ( -64.00000000000045475, -7.632783294297951215E-14, -2.000000000000001776 ) ) ;
#4720=DIRECTION ( 'NONE',  ( 0.000000000000000000, 0.000000000000000000, -1.000000000000000000 ) ) ;
#4726=ORIENTED_EDGE ( 'NONE', *, *, #5664, .T. ) ;
#4731=DIRECTION ( 'NONE',  ( 1.000000000000000000, 1.479114197289388027E-30, -2.013525853228518840E-32 ) ) ;
#4741=PLANE ( 'NONE',  #15173 ) ;
#4743=ADVANCED_FACE ( 'NONE', ( #3279 ), #6927, .T. ) ;
#4744=DIRECTION ( 'NONE',  ( -2.220446049250313081E-16, 1.000000000000000000, -7.025792437124636392E-31 ) ) ;
#4746=CARTESIAN_POINT ( 'NONE',  ( -43.10883117545714782, -4.565685424949276872, 7.500000000000062172 ) ) ;
#4754=ORIENTED_EDGE ( 'NONE', *, *, #5134, .T. ) ;
#4755=VERTEX_POINT ( 'NONE', #11764 ) ;
#4758=EDGE_LOOP ( 'NONE', ( #14700, #2295 ) ) ;
#4759=LINE ( 'NONE', #16980, #19697 ) ;
#4774=ORIENTED_EDGE ( 'NONE', *, *, #2601, .F. ) ;
#4784=EDGE_CURVE ( 'NONE', #13378, #18638, #17108, .T. ) ;
#4786=CARTESIAN_POINT ( 'NONE',  ( -50.65685424949275983, 7.200000000000018829, -8.000000000000007105 ) ) ;
#4788=ORIENTED_EDGE ( 'NONE', *, *, #12520, .T. ) ;
#4804=DIRECTION ( 'NONE',  ( -2.013525853228507892E-32, -6.902532920683810383E-31, 1.000000000000000000 ) ) ;
#4806=DIRECTION ( 'NONE',  ( 2.013525853228507892E-32, 6.902532920683810383E-31, -1.000000000000000000 ) ) ;
#4818=CARTESIAN_POINT ( 'NONE',  ( -89.70000000000064233, 5.551115123125782702E-14, -2.000000000000001776 ) ) ;
#4821=DIRECTION ( 'NONE',  ( 2.013525853228507892E-32, 6.902532920683810383E-31, -1.000000000000000000 ) ) ;
#4822=DIRECTION ( 'NONE',  ( -0.7071067811865490160, -0.7071067811865460184, -1.565905175853766674E-16 ) ) ;
#4824=PLANE ( 'NONE',  #6878 ) ;
#4826=CARTESIAN_POINT ( 'NONE',  ( -6.000000000000130562, 7.999999999999958256, -8.000000000000035527 ) ) ;
#4827=CARTESIAN_POINT ( 'NONE',  ( -67.40537636629493079, 0.5000000000000143219, 12.70639812373644517 ) ) ;
#4828=DIRECTION ( 'NONE',  ( -2.220446049250313081E-16, 1.000000000000000000, -7.025792437124636392E-31 ) ) ;
#4829=EDGE_CURVE ( 'NONE', #17901, #13088, #5482, .T. ) ;
#4831=AXIS2_PLACEMENT_3D ( 'NONE', #13025, #2308, #11019 ) ;
#4840=ADVANCED_FACE ( 'NONE', ( #21515 ), #7496, .T. ) ;
#4849=DIRECTION ( 'NONE',  ( 2.013525853228507892E-32, 6.902532920683810383E-31, -1.000000000000000000 ) ) ;
#4851=CARTESIAN_POINT ( 'NONE',  ( -6.000000000000102141, 5.299999999999964295, 8.000000000000047962 ) ) ;
#4855=( NAMED_UNIT ( * ) SI_UNIT ( $, .STERADIAN. ) SOLID_ANGLE_UNIT ( ) );
#4861=ORIENTED_EDGE ( 'NONE', *, *, #11822, .T. ) ;
#4862=VERTEX_POINT ( 'NONE', #436 ) ;
#4865=AXIS2_PLACEMENT_3D ( 'NONE', #3366, #17693, #6887 ) ;
#4866=ORIENTED_EDGE ( 'NONE', *, *, #22624, .F. ) ;
#4868=ORIENTED_EDGE ( 'NONE', *, *, #17260, .F. ) ;
#4883=LINE ( 'NONE', #9010, #11784 ) ;
#4886=CARTESIAN_POINT ( 'NONE',  ( -6.000000000000143885, -2.000000000000043521, -8.000000000000035527 ) ) ;
#4887=VERTEX_POINT ( 'NONE', #10895 ) ;
#4893=DIRECTION ( 'NONE',  ( -2.013525853228507892E-32, -6.902532920683810383E-31, 1.000000000000000000 ) ) ;
#4898=CARTESIAN_POINT ( 'NONE',  ( -42.54314575050785407, -8.000000000000000000, -7.500000000000007105 ) ) ;
#4915=VECTOR ( 'NONE', #326, 1000.000000000000000 ) ;
#4918=ADVANCED_FACE ( 'NONE', ( #6400 ), #18210, .T. ) ;
#4923=ORIENTED_EDGE ( 'NONE', *, *, #16684, .F. ) ;
#4936=DIRECTION ( 'NONE',  ( 2.013525853228507892E-32, 6.902532920683810383E-31, -1.000000000000000000 ) ) ;
#4943=CARTESIAN_POINT ( 'NONE',  ( 0.000000000000000000, 0.000000000000000000, 0.000000000000000000 ) ) ;
#4947=CIRCLE ( 'NONE', #5726, 3.500000000000023981 ) ;
#4950=ORIENTED_EDGE ( 'NONE', *, *, #9950, .F. ) ;
#4951=ORIENTED_EDGE ( 'NONE', *, *, #15535, .T. ) ;
#4954=CARTESIAN_POINT ( 'NONE',  ( -42.54314575050793934, -8.000000000000021316, 7.500000000000062172 ) ) ;
#4955=CARTESIAN_POINT ( 'NONE',  ( -50.65685424949273141, 7.200000000000025935, 8.000000000000076383 ) ) ;
#4958=( GEOMETRIC_REPRESENTATION_CONTEXT ( 3 ) GLOBAL_UNCERTAINTY_ASSIGNED_CONTEXT ( ( #16374 ) ) GLOBAL_UNIT_ASSIGNED_CONTEXT ( ( #6176, #876, #4855 ) ) REPRESENTATION_CONTEXT ( 'NONE', 'WORKASPACE' ) );
#4967=AXIS2_PLACEMENT_3D ( 'NONE', #19036, #13272, #8326 ) ;
#4979=ORIENTED_EDGE ( 'NONE', *, *, #21482, .F. ) ;
#4986=CIRCLE ( 'NONE', #12887, 0.5000000000000006661 ) ;
#4987=VECTOR ( 'NONE', #8305, 1000.000000000000000 ) ;
#4995=DIRECTION ( 'NONE',  ( 1.000000000000000000, -1.365024226554777580E-62, 2.013525853228508439E-32 ) ) ;
#4997=FACE_OUTER_BOUND ( 'NONE', #20249, .T. ) ;
#5006=ORIENTED_EDGE ( 'NONE', *, *, #8339, .T. ) ;
#5014=ORIENTED_EDGE ( 'NONE', *, *, #10214, .T. ) ;
#5019=VECTOR ( 'NONE', #14899, 1000.000000000000000 ) ;
#5031=CARTESIAN_POINT ( 'NONE',  ( -6.000000000000088818, -2.000000000000043521, 7.500000000000076383 ) ) ;
#5055=ORIENTED_EDGE ( 'NONE', *, *, #16336, .F. ) ;
#5061=DIRECTION ( 'NONE',  ( -1.000000000000000000, 1.365024226554778012E-62, -2.013525853228508439E-32 ) ) ;
#5065=DIRECTION ( 'NONE',  ( 2.220446049250313081E-16, -1.000000000000000000, 7.025792437124636392E-31 ) ) ;
#5073=ORIENTED_EDGE ( 'NONE', *, *, #21177, .T. ) ;
#5074=AXIS2_PLACEMENT_3D ( 'NONE', #21045, #23045, #10678 ) ;
#5077=VERTEX_POINT ( 'NONE', #10417 ) ;
#5078=ORIENTED_EDGE ( 'NONE', *, *, #3455, .F. ) ;
#5082=EDGE_CURVE ( 'NONE', #23028, #13536, #19717, .T. ) ;
#5083=ORIENTED_EDGE ( 'NONE', *, *, #3509, .F. ) ;
#5087=CARTESIAN_POINT ( 'NONE',  ( -0.5000000000000975886, 1.999999999999890754, 7.500000000000007105 ) ) ;
#5092=DIRECTION ( 'NONE',  ( 1.550910762415566494E-16, 1.000000000000000000, -8.135128085091684243E-31 ) ) ;
#5096=FACE_OUTER_BOUND ( 'NONE', #20280, .T. ) ;
#5098=EDGE_CURVE ( 'NONE', #9917, #11317, #9118, .T. ) ;
#5105=VERTEX_POINT ( 'NONE', #18289 ) ;
#5106=EDGE_CURVE ( 'NONE', #5668, #8762, #11141, .T. ) ;
#5110=EDGE_LOOP ( 'NONE', ( #13789, #10488, #14536, #1486 ) ) ;
#5115=CARTESIAN_POINT ( 'NONE',  ( -50.65685424949274562, 7.200000000000025935, 17.71251237973613257 ) ) ;
#5119=CARTESIAN_POINT ( 'NONE',  ( -95.70000000000069917, 2.700000000000014833, -2.000000000000001776 ) ) ;
#5121=PLANE ( 'NONE',  #4572 ) ;
#5128=AXIS2_PLACEMENT_3D ( 'NONE', #9, #119, #21422 ) ;
#5134=EDGE_CURVE ( 'NONE', #1775, #1329, #21301, .T. ) ;
#5144=CARTESIAN_POINT ( 'NONE',  ( -42.54314575050793934, 7.999999999999992895, 8.000000000000035527 ) ) ;
#5145=LINE ( 'NONE', #17368, #7965 ) ;
#5147=DIRECTION ( 'NONE',  ( 2.013525853228507892E-32, 6.902532920683810383E-31, -1.000000000000000000 ) ) ;
#5151=AXIS2_PLACEMENT_3D ( 'NONE', #9559, #13976, #22496 ) ;
#5157=DIRECTION ( 'NONE',  ( 0.000000000000000000, 0.000000000000000000, -1.000000000000000000 ) ) ;
#5162=ORIENTED_EDGE ( 'NONE', *, *, #2459, .F. ) ;
#5165=AXIS2_PLACEMENT_3D ( 'NONE', #3846, #21855, #5866 ) ;
#5171=CARTESIAN_POINT ( 'NONE',  ( -55.05572809000125289, 0.5000000000000143219, -10.00000000000006395 ) ) ;
#5174=CARTESIAN_POINT ( 'NONE',  ( -42.54314575050793934, -4.000000000000021316, 7.500000000000062172 ) ) ;
#5176=EDGE_LOOP ( 'NONE', ( #3821, #21811, #2583, #6844 ) ) ;
#5181=CARTESIAN_POINT ( 'NONE',  ( -6.000000000000047073, -4.800000000000006040, 8.000000000000090594 ) ) ;
#5183=CARTESIAN_POINT ( 'NONE',  ( -42.54314575050785407, -4.000000000000021316, 8.000000000000007105 ) ) ;
#5185=LINE ( 'NONE', #10922, #8387 ) ;
#5186=DIRECTION ( 'NONE',  ( -1.550910762415566494E-16, -1.000000000000000000, 8.135128085091684243E-31 ) ) ;
#5218=VECTOR ( 'NONE', #6349, 1000.000000000000000 ) ;
#5223=ADVANCED_FACE ( 'NONE', ( #11227 ), #5942, .T. ) ;
#5225=EDGE_CURVE ( 'NONE', #12501, #4139, #6288, .T. ) ;
#5227=CARTESIAN_POINT ( 'NONE',  ( -95.70000000000071338, 2.700000000000014833, 1.000000000000070166 ) ) ;
#5228=ORIENTED_EDGE ( 'NONE', *, *, #12419, .F. ) ;
#5229=ORIENTED_EDGE ( 'NONE', *, *, #752, .F. ) ;
#5231=VECTOR ( 'NONE', #22717, 1000.000000000000114 ) ;
#5240=ADVANCED_FACE ( 'NONE', ( #16618 ), #13222, .T. ) ;
#5244=EDGE_LOOP ( 'NONE', ( #16892, #23237 ) ) ;
#5245=CARTESIAN_POINT ( 'NONE',  ( -65.00000000000046896, -0.5000000000000628386, 3.000000000000030198 ) ) ;
#5248=CARTESIAN_POINT ( 'NONE',  ( -65.55642023346347003, -0.5000000000000628386, -11.87813525200320797 ) ) ;
#5253=DIRECTION ( 'NONE',  ( -1.000000000000000000, -6.938893903907186568E-15, 0.000000000000000000 ) ) ;
#5273=DIRECTION ( 'NONE',  ( 2.013525853228507892E-32, 6.902532920683810383E-31, -1.000000000000000000 ) ) ;
#5275=CARTESIAN_POINT ( 'NONE',  ( -3.200000000000091660, 5.299999999999998934, -8.000000000000035527 ) ) ;
#5276=DIRECTION ( 'NONE',  ( -2.013525853228507892E-32, -6.902532920683810383E-31, 1.000000000000000000 ) ) ;
#5278=DIRECTION ( 'NONE',  ( 1.550910762415566494E-16, 1.000000000000000000, -8.135128085091684243E-31 ) ) ;
#5280=CARTESIAN_POINT ( 'NONE',  ( -89.70000000000048601, -2.700000000000084110, 1.000000000000000888 ) ) ;
#5284=TOROIDAL_SURFACE ( 'NONE', #3034, 6.700000000000001066, 0.5000000000000000000 ) ;
#5285=ORIENTED_EDGE ( 'NONE', *, *, #4036, .T. ) ;
#5291=FACE_OUTER_BOUND ( 'NONE', #14629, .T. ) ;
#5297=CARTESIAN_POINT ( 'NONE',  ( -6.000000000000116351, 1.999999999999960032, -7.500000000000062172 ) ) ;
#5299=LINE ( 'NONE', #19886, #5557 ) ;
#5304=MANIFOLD_SOLID_BREP ( 'Fillet1', #14061 ) ;
#5306=DIRECTION ( 'NONE',  ( 1.000000000000000000, 0.000000000000000000, 0.000000000000000000 ) ) ;
#5307=ORIENTED_EDGE ( 'NONE', *, *, #14027, .F. ) ;
#5311=ADVANCED_FACE ( 'NONE', ( #5096 ), #3477, .T. ) ;
#5324=DIRECTION ( 'NONE',  ( -1.000000000000000000, 1.550910762415526064E-16, 0.000000000000000000 ) ) ;
#5325=DIRECTION ( 'NONE',  ( 1.000000000000000000, 0.000000000000000000, 0.000000000000000000 ) ) ;
#5335=LINE ( 'NONE', #15789, #2509 ) ;
#5350=LINE ( 'NONE', #22888, #17427 ) ;
#5364=CARTESIAN_POINT ( 'NONE',  ( -67.28510754798023186, 2.700000000000021938, 12.22107821754961421 ) ) ;
#5375=EDGE_LOOP ( 'NONE', ( #13847, #10335, #11434, #6875 ) ) ;
#5380=ORIENTED_EDGE ( 'NONE', *, *, #586, .F. ) ;
#5384=VERTEX_POINT ( 'NONE', #19439 ) ;
#5392=DIRECTION ( 'NONE',  ( 1.000000000000000000, 2.168404344970991858E-16, 5.348730717595112872E-15 ) ) ;
#5396=CARTESIAN_POINT ( 'NONE',  ( -47.47487373415321343, -4.018019484660590557, 7.500000000000062172 ) ) ;
#5397=VECTOR ( 'NONE', #10147, 1000.000000000000000 ) ;
#5405=EDGE_LOOP ( 'NONE', ( #17117, #20813, #1067, #4675 ) ) ;
#5409=CIRCLE ( 'NONE', #10649, 4.000000000000023981 ) ;
#5413=DIRECTION ( 'NONE',  ( -2.013525853228507892E-32, -6.902532920683810383E-31, 1.000000000000000000 ) ) ;
#5424=LINE ( 'NONE', #1868, #15791 ) ;
#5425=LINE ( 'NONE', #3648, #3138 ) ;
#5431=AXIS2_PLACEMENT_3D ( 'NONE', #18886, #22184, #6069 ) ;
#5434=SHAPE_DEFINITION_REPRESENTATION ( #19249, #20536 ) ;
#5438=VERTEX_POINT ( 'NONE', #9206 ) ;
#5451=DIRECTION ( 'NONE',  ( -0.9706398123736329486, 1.505375731439247187E-16, -0.2405376366294442458 ) ) ;
#5452=DIRECTION ( 'NONE',  ( -1.000000000000000000, 1.369518533665891191E-16, -1.780374093765658523E-15 ) ) ;
#5460=ORIENTED_EDGE ( 'NONE', *, *, #22711, .F. ) ;
#5462=EDGE_LOOP ( 'NONE', ( #12391, #3575 ) ) ;
#5463=ORIENTED_EDGE ( 'NONE', *, *, #21283, .T. ) ;
#5468=ORIENTED_EDGE ( 'NONE', *, *, #10075, .F. ) ;
#5470=LINE ( 'NONE', #5929, #10298 ) ;
#5472=CIRCLE ( 'NONE', #6224, 4.000000000000023981 ) ;
#5479=DIRECTION ( 'NONE',  ( -1.550910762415566494E-16, -1.000000000000000000, 8.135128085091684243E-31 ) ) ;
#5482=CIRCLE ( 'NONE', #13740, 0.5000000000000039968 ) ;
#5483=CARTESIAN_POINT ( 'NONE',  ( -6.000000000000116351, 1.999999999999960032, -7.500000000000062172 ) ) ;
#5495=AXIS2_PLACEMENT_3D ( 'NONE', #8462, #22702, #20831 ) ;
#5508=VECTOR ( 'NONE', #21760, 1000.000000000000000 ) ;
#5509=CARTESIAN_POINT ( 'NONE',  ( -55.05572809000125289, -1.040834085586084257E-13, -10.00000000000006395 ) ) ;
#5536=DIRECTION ( 'NONE',  ( -2.013525853228507892E-32, -6.902532920683810383E-31, 1.000000000000000000 ) ) ;
#5538=DIRECTION ( 'NONE',  ( 0.7071067811865524577, 0.7071067811865425767, 2.121016688166341246E-16 ) ) ;
#5545=ORIENTED_EDGE ( 'NONE', *, *, #10091, .F. ) ;
#5550=TOROIDAL_SURFACE ( 'NONE', #21346, 9.499999999999998224, 0.5000000000000000000 ) ;
#5557=VECTOR ( 'NONE', #12585, 1000.000000000000000 ) ;
#5578=ORIENTED_EDGE ( 'NONE', *, *, #20728, .T. ) ;
#5588=ORIENTED_EDGE ( 'NONE', *, *, #16336, .T. ) ;
#5598=FACE_OUTER_BOUND ( 'NONE', #394, .T. ) ;
#5604=AXIS2_PLACEMENT_3D ( 'NONE', #9429, #2248, #9546 ) ;
#5607=TOROIDAL_SURFACE ( 'NONE', #22879, 5.500000000000003553, 0.5000000000000000000 ) ;
#5611=ORIENTED_EDGE ( 'NONE', *, *, #10211, .T. ) ;
#5613=ORIENTED_EDGE ( 'NONE', *, *, #3838, .T. ) ;
#5619=DIRECTION ( 'NONE',  ( 0.7071067811865233699, -0.7071067811865715536, -1.565905175853783930E-16 ) ) ;
#5632=DIRECTION ( 'NONE',  ( 1.000000000000000000, 2.220446049250313081E-16, -3.656342123407315983E-48 ) ) ;
#5633=ORIENTED_EDGE ( 'NONE', *, *, #15869, .T. ) ;
#5635=ORIENTED_EDGE ( 'NONE', *, *, #16023, .T. ) ;
#5637=DIRECTION ( 'NONE',  ( -1.000000000000000000, 1.550910762415506096E-16, 0.000000000000000000 ) ) ;
#5639=VERTEX_POINT ( 'NONE', #6140 ) ;
#5640=VECTOR ( 'NONE', #20288, 1000.000000000000000 ) ;
#5649=ADVANCED_FACE ( 'NONE', ( #17407 ), #9901, .T. ) ;
#5651=DIRECTION ( 'NONE',  ( 2.013525853219271912E-32, -5.941108692445745160E-30, -1.000000000000000000 ) ) ;
#5655=CARTESIAN_POINT ( 'NONE',  ( -42.54314575050785407, -8.000000000000021316, 8.000000000000007105 ) ) ;
#5656=DIRECTION ( 'NONE',  ( -0.1556420233463076119, 0.000000000000000000, -0.9878135252003121813 ) ) ;
#5661=EDGE_CURVE ( 'NONE', #6467, #15244, #19253, .T. ) ;
#5663=EDGE_CURVE ( 'NONE', #22523, #7574, #15412, .T. ) ;
#5664=EDGE_CURVE ( 'NONE', #9669, #12565, #2840, .T. ) ;
#5666=EDGE_LOOP ( 'NONE', ( #3550, #2113, #3921, #10997 ) ) ;
#5668=VERTEX_POINT ( 'NONE', #4827 ) ;
#5669=ORIENTED_EDGE ( 'NONE', *, *, #586, .T. ) ;
#5676=CARTESIAN_POINT ( 'NONE',  ( -47.47487373415326317, 4.018019484660594109, -7.500000000000034639 ) ) ;
#5689=VERTEX_POINT ( 'NONE', #8362 ) ;
#5691=CIRCLE ( 'NONE', #10190, 0.5000000000000029976 ) ;
#5694=ORIENTED_EDGE ( 'NONE', *, *, #21040, .F. ) ;
#5701=EDGE_CURVE ( 'NONE', #17530, #4755, #16460, .T. ) ;
#5704=ORIENTED_EDGE ( 'NONE', *, *, #20698, .T. ) ;
#5707=LINE ( 'NONE', #19940, #7161 ) ;
#5711=CARTESIAN_POINT ( 'NONE',  ( -43.06238456605046849, 5.319238815542546739, -7.499999999999978684 ) ) ;
#5721=ORIENTED_EDGE ( 'NONE', *, *, #15099, .T. ) ;
#5723=ORIENTED_EDGE ( 'NONE', *, *, #11203, .T. ) ;
#5724=EDGE_LOOP ( 'NONE', ( #13360, #17359, #6595, #17186, #21188, #1641, #4570, #11893, #11633, #18768, #10715, #13351 ) ) ;
#5726=AXIS2_PLACEMENT_3D ( 'NONE', #17134, #18804, #16669 ) ;
#5728=CIRCLE ( 'NONE', #7650, 6.700000000000039257 ) ;
#5731=CARTESIAN_POINT ( 'NONE',  ( -87.15000000000055991, -3.200000000000092104, -2.000000000000002220 ) ) ;
#5740=CIRCLE ( 'NONE', #1240, 0.5000000000000029976 ) ;
#5745=VECTOR ( 'NONE', #11128, 1000.000000000000000 ) ;
#5746=EDGE_CURVE ( 'NONE', #21208, #22909, #2946, .T. ) ;
#5751=CYLINDRICAL_SURFACE ( 'NONE', #18513, 0.5000000000000025535 ) ;
#5756=CIRCLE ( 'NONE', #21551, 6.000000000000036415 ) ;
#5758=DIRECTION ( 'NONE',  ( -2.220446049250313081E-16, 1.000000000000000000, -7.025792437124636392E-31 ) ) ;
#5760=CARTESIAN_POINT ( 'NONE',  ( -45.91923881554271958, -2.462384566050183743, -7.500000000000034639 ) ) ;
#5761=CIRCLE ( 'NONE', #8758, 5.500000000000032863 ) ;
#5778=CIRCLE ( 'NONE', #10282, 9.500000000000056843 ) ;
#5786=ORIENTED_EDGE ( 'NONE', *, *, #2102, .T. ) ;
#5787=PLANE ( 'NONE',  #9904 ) ;
#5791=ORIENTED_EDGE ( 'NONE', *, *, #6119, .F. ) ;
#5796=CARTESIAN_POINT ( 'NONE',  ( -45.37157287525410254, 6.828427124746169419, 8.000000000000035527 ) ) ;
#5798=EDGE_CURVE ( 'NONE', #19780, #6327, #4063, .T. ) ;
#5807=ADVANCED_FACE ( 'NONE', ( #7310 ), #10479, .T. ) ;
#5815=CIRCLE ( 'NONE', #2418, 9.500000000000063949 ) ;
#5817=VERTEX_POINT ( 'NONE', #6964 ) ;
#5846=ORIENTED_EDGE ( 'NONE', *, *, #17002, .T. ) ;
#5847=ORIENTED_EDGE ( 'NONE', *, *, #10877, .T. ) ;
#5852=CARTESIAN_POINT ( 'NONE',  ( -53.99613665484950786, 1.387778780781445676E-14, -13.19342998475048212 ) ) ;
#5856=DIRECTION ( 'NONE',  ( 2.220446049250313081E-16, -1.000000000000000000, 7.025792437124636392E-31 ) ) ;
#5857=CARTESIAN_POINT ( 'NONE',  ( -90.63385214007844581, 0.5000000000000490719, -7.926881151201908615 ) ) ;
#5866=DIRECTION ( 'NONE',  ( 1.000000000000000000, 1.479114197289387852E-30, -2.013525853228518840E-32 ) ) ;
#5875=DIRECTION ( 'NONE',  ( -2.220446049250313081E-16, 1.000000000000000000, -7.025792437124636392E-31 ) ) ;
#5876=DIRECTION ( 'NONE',  ( -1.000000000000000000, 1.550910762415518915E-16, 0.000000000000000000 ) ) ;
#5878=PLANE ( 'NONE',  #12058 ) ;
#5882=CARTESIAN_POINT ( 'NONE',  ( -45.56568542494955665, 2.108831175456925333, -7.500000000000007105 ) ) ;
#5883=ORIENTED_EDGE ( 'NONE', *, *, #14900, .F. ) ;
#5884=DIRECTION ( 'NONE',  ( 0.9878135252003128475, 2.193386639427060968E-16, -0.1556420233463030045 ) ) ;
#5889=CIRCLE ( 'NONE', #10755, 0.5000000000000028866 ) ;
#5890=ORIENTED_EDGE ( 'NONE', *, *, #18762, .T. ) ;
#5892=DIRECTION ( 'NONE',  ( -1.000000000000000000, 1.813574543066650990E-15, 0.000000000000000000 ) ) ;
#5894=ADVANCED_FACE ( 'NONE', ( #21311 ), #131, .F. ) ;
#5897=FACE_OUTER_BOUND ( 'NONE', #20595, .T. ) ;
#5912=ORIENTED_EDGE ( 'NONE', *, *, #20442, .T. ) ;
#5916=ORIENTED_EDGE ( 'NONE', *, *, #21499, .T. ) ;
#5921=VERTEX_POINT ( 'NONE', #10589 ) ;
#5929=CARTESIAN_POINT ( 'NONE',  ( -95.70000000000069917, 2.775557561562891351E-14, -2.000000000000001776 ) ) ;
#5933=DIRECTION ( 'NONE',  ( -1.000000000000000000, -1.110223024625164429E-16, 1.298062744027674633E-32 ) ) ;
#5938=DIRECTION ( 'NONE',  ( 1.000000000000000000, 2.220446049250313081E-16, 0.000000000000000000 ) ) ;
#5942=CYLINDRICAL_SURFACE ( 'NONE', #1575, 10.00000000000006395 ) ;
#5948=ORIENTED_EDGE ( 'NONE', *, *, #19313, .F. ) ;
#5951=EDGE_LOOP ( 'NONE', ( #8577, #1635, #3153, #489 ) ) ;
#5975=CYLINDRICAL_SURFACE ( 'NONE', #10845, 0.5000000000000038858 ) ;
#5981=ORIENTED_EDGE ( 'NONE', *, *, #6239, .T. ) ;
#5985=AXIS2_PLACEMENT_3D ( 'NONE', #18523, #12767, #7708 ) ;
#5986=DIRECTION ( 'NONE',  ( 1.000000000000000000, -1.424116703980815236E-16, -2.931272055834072749E-32 ) ) ;
#5988=VECTOR ( 'NONE', #19020, 1000.000000000000000 ) ;
#5989=CIRCLE ( 'NONE', #19126, 0.5000000000000004441 ) ;
#5995=CARTESIAN_POINT ( 'NONE',  ( -42.54314575050793934, 3.999999999999996447, 7.500000000000062172 ) ) ;
#6003=CARTESIAN_POINT ( 'NONE',  ( -42.54314575050796776, 4.800000000000033573, -8.000000000000035527 ) ) ;
#6011=ORIENTED_EDGE ( 'NONE', *, *, #6078, .T. ) ;
#6013=DIRECTION ( 'NONE',  ( -2.013525853228508439E-32, -6.779273404243028164E-31, 1.000000000000000000 ) ) ;
#6014=CARTESIAN_POINT ( 'NONE',  ( -50.65685424949270299, 7.200000000000025935, 7.500000000000062172 ) ) ;
#6016=ORIENTED_EDGE ( 'NONE', *, *, #12772, .T. ) ;
#6023=AXIS2_PLACEMENT_3D ( 'NONE', #21987, #5875, #20229 ) ;
#6024=CARTESIAN_POINT ( 'NONE',  ( -50.65685424949277404, -1.040834085586084257E-13, -7.500000000000062172 ) ) ;
#6035=ORIENTED_EDGE ( 'NONE', *, *, #484, .T. ) ;
#6038=ORIENTED_EDGE ( 'NONE', *, *, #10119, .T. ) ;
#6051=CARTESIAN_POINT ( 'NONE',  ( -89.70000000000059970, 4.857225732735059864E-14, 1.000000000000000888 ) ) ;
#6054=EDGE_CURVE ( 'NONE', #4755, #5817, #329, .T. ) ;
#6058=CARTESIAN_POINT ( 'NONE',  ( -45.37157287525410254, 6.828427124746163202, 8.000000000000035527 ) ) ;
#6069=DIRECTION ( 'NONE',  ( 1.000000000000000000, 1.240809152955624894E-14, 0.000000000000000000 ) ) ;
#6070=AXIS2_PLACEMENT_3D ( 'NONE', #11134, #103, #7608 ) ;
#6076=FACE_OUTER_BOUND ( 'NONE', #6536, .T. ) ;
#6078=EDGE_CURVE ( 'NONE', #6815, #17750, #2689, .T. ) ;
#6081=EDGE_CURVE ( 'NONE', #14457, #21664, #3661, .T. ) ;
#6088=ORIENTED_EDGE ( 'NONE', *, *, #3455, .T. ) ;
#6095=ORIENTED_EDGE ( 'NONE', *, *, #13415, .F. ) ;
#6103=ORIENTED_EDGE ( 'NONE', *, *, #18215, .T. ) ;
#6107=LINE ( 'NONE', #19041, #22084 ) ;
#6109=CIRCLE ( 'NONE', #21886, 6.700000000000039257 ) ;
#6119=EDGE_CURVE ( 'NONE', #3000, #13876, #11865, .T. ) ;
#6122=ORIENTED_EDGE ( 'NONE', *, *, #10639, .F. ) ;
#6123=AXIS2_PLACEMENT_3D ( 'NONE', #16038, #19466, #23001 ) ;
#6124=CIRCLE ( 'NONE', #4598, 5.500000000000032863 ) ;
#6125=ORIENTED_EDGE ( 'NONE', *, *, #227, .T. ) ;
#6126=EDGE_LOOP ( 'NONE', ( #14854, #5890, #11293, #9191 ) ) ;
#6128=DIRECTION ( 'NONE',  ( 1.000000000000000000, 1.479114197289388027E-30, -2.013525853228518840E-32 ) ) ;
#6132=CYLINDRICAL_SURFACE ( 'NONE', #9794, 0.5000000000000028866 ) ;
#6136=VECTOR ( 'NONE', #10791, 1000.000000000000000 ) ;
#6140=CARTESIAN_POINT ( 'NONE',  ( -50.65685424949275983, -2.700000000000091216, -8.000000000000007105 ) ) ;
#6141=CIRCLE ( 'NONE', #10631, 9.500000000000063949 ) ;
#6143=AXIS2_PLACEMENT_3D ( 'NONE', #10007, #11292, #18598 ) ;
#6148=CARTESIAN_POINT ( 'NONE',  ( -56.91911807125104872, -0.5000000000001045830, -8.333333333333413862 ) ) ;
#6151=ORIENTED_EDGE ( 'NONE', *, *, #17910, .T. ) ;
#6158=ORIENTED_EDGE ( 'NONE', *, *, #11836, .F. ) ;
#6159=CIRCLE ( 'NONE', #19295, 3.300000000000019806 ) ;
#6160=EDGE_LOOP ( 'NONE', ( #9792, #225, #10393, #5883 ) ) ;
#6163=AXIS2_PLACEMENT_3D ( 'NONE', #16300, #12896, #14888 ) ;
#6169=DIRECTION ( 'NONE',  ( -1.000000000000000000, 1.389842848855773367E-62, -2.013525853228507892E-32 ) ) ;
#6176=( LENGTH_UNIT ( ) NAMED_UNIT ( * ) SI_UNIT ( .MILLI., .METRE. ) );
#6180=DIRECTION ( 'NONE',  ( 2.220446049250313081E-16, -1.000000000000000000, 7.025792437124636392E-31 ) ) ;
#6186=ORIENTED_EDGE ( 'NONE', *, *, #20019, .T. ) ;
#6193=CARTESIAN_POINT ( 'NONE',  ( -6.000000000000088818, -2.000000000000043521, 7.500000000000076383 ) ) ;
#6207=AXIS2_PLACEMENT_3D ( 'NONE', #20111, #9633, #22224 ) ;
#6221=CARTESIAN_POINT ( 'NONE',  ( -0.5000000000000837108, 1.999999999999890754, 8.000000000000076383 ) ) ;
#6224=AXIS2_PLACEMENT_3D ( 'NONE', #6014, #11522, #13416 ) ;
#6236=DIRECTION ( 'NONE',  ( -2.220446049250313081E-16, 1.000000000000000000, -7.025792437124636392E-31 ) ) ;
#6239=EDGE_CURVE ( 'NONE', #4603, #4887, #20196, .T. ) ;
#6243=VERTEX_POINT ( 'NONE', #1736 ) ;
#6248=EDGE_LOOP ( 'NONE', ( #17651, #13815, #9537, #4 ) ) ;
#6261=DIRECTION ( 'NONE',  ( -2.013525853228507892E-32, -6.902532920683810383E-31, 1.000000000000000000 ) ) ;
#6263=LINE ( 'NONE', #13198, #12269 ) ;
#6268=CIRCLE ( 'NONE', #2118, 0.5000000000000004441 ) ;
#6277=VECTOR ( 'NONE', #18742, 1000.000000000000000 ) ;
#6288=LINE ( 'NONE', #2402, #20751 ) ;
#6289=EDGE_CURVE ( 'NONE', #18669, #10966, #10411, .T. ) ;
#6300=ORIENTED_EDGE ( 'NONE', *, *, #8934, .F. ) ;
#6301=AXIS2_PLACEMENT_3D ( 'NONE', #2902, #6438, #13498 ) ;
#6311=CARTESIAN_POINT ( 'NONE',  ( -50.65685424949277404, 3.200000000000022382, 8.000000000000021316 ) ) ;
#6318=DIRECTION ( 'NONE',  ( -1.000000000000000000, 1.337182679398780230E-14, 0.000000000000000000 ) ) ;
#6320=CARTESIAN_POINT ( 'NONE',  ( -6.000000000000143885, 1.999999999999960032, 8.000000000000062172 ) ) ;
#6321=DIRECTION ( 'NONE',  ( -1.000000000000000000, -1.479114197289388027E-30, 2.013525853228518840E-32 ) ) ;
#6327=VERTEX_POINT ( 'NONE', #27 ) ;
#6338=DIRECTION ( 'NONE',  ( -1.000000000000000000, 1.550910762415513985E-16, 3.012982189080959477E-32 ) ) ;
#6348=CARTESIAN_POINT ( 'NONE',  ( -1.249000902703301108E-13, -6.938893903907228378E-14, 8.000000000000062172 ) ) ;
#6349=DIRECTION ( 'NONE',  ( 2.013525853228507892E-32, 6.902532920683810383E-31, -1.000000000000000000 ) ) ;
#6350=EDGE_CURVE ( 'NONE', #3000, #17067, #13051, .T. ) ;
#6355=VECTOR ( 'NONE', #13252, 1000.000000000000114 ) ;
#6360=EDGE_CURVE ( 'NONE', #15244, #5077, #3285, .T. ) ;
#6368=CARTESIAN_POINT ( 'NONE',  ( -3.200000000000091660, -2.000000000000050182, -7.500000000000034639 ) ) ;
#6378=ADVANCED_FACE ( 'NONE', ( #21851 ), #3841, .T. ) ;
#6379=EDGE_CURVE ( 'NONE', #7024, #9098, #9813, .T. ) ;
#6385=ORIENTED_EDGE ( 'NONE', *, *, #10223, .F. ) ;
#6398=CARTESIAN_POINT ( 'NONE',  ( -55.25320565519148630, -2.775557561562891351E-14, 7.500000000000007105 ) ) ;
#6399=DIRECTION ( 'NONE',  ( 2.220446049250313081E-16, -1.000000000000000000, 7.025792437124636392E-31 ) ) ;
#6400=FACE_OUTER_BOUND ( 'NONE', #23021, .T. ) ;
#6401=CARTESIAN_POINT ( 'NONE',  ( -6.000000000000116351, 7.999999999999958256, -7.500000000000062172 ) ) ;
#6405=CARTESIAN_POINT ( 'NONE',  ( -6.000000000000074607, 7.999999999999958256, 7.500000000000062172 ) ) ;
#6412=AXIS2_PLACEMENT_3D ( 'NONE', #6619, #10263, #15779 ) ;
#6415=ADVANCED_FACE ( 'NONE', ( #20764 ), #13804, .T. ) ;
#6436=ORIENTED_EDGE ( 'NONE', *, *, #9672, .F. ) ;
#6438=DIRECTION ( 'NONE',  ( -2.013525853228507892E-32, -6.902532920683810383E-31, 1.000000000000000000 ) ) ;
#6454=CARTESIAN_POINT ( 'NONE',  ( -42.54314575050799618, 3.999999999999996447, 8.000000000000035527 ) ) ;
#6466=VERTEX_POINT ( 'NONE', #2081 ) ;
#6467=VERTEX_POINT ( 'NONE', #19969 ) ;
#6471=LINE ( 'NONE', #8241, #12593 ) ;
#6475=DIRECTION ( 'NONE',  ( 0.000000000000000000, 0.000000000000000000, 1.000000000000000000 ) ) ;
#6478=ADVANCED_FACE ( 'NONE', ( #7503 ), #5550, .T. ) ;
#6492=VERTEX_POINT ( 'NONE', #3229 ) ;
#6493=VECTOR ( 'NONE', #22442, 1000.000000000000114 ) ;
#6511=DIRECTION ( 'NONE',  ( 1.000000000000000000, 0.000000000000000000, 0.000000000000000000 ) ) ;
#6512=VECTOR ( 'NONE', #3213, 1000.000000000000000 ) ;
#6513=ADVANCED_FACE ( 'NONE', ( #10506 ), #3106, .T. ) ;
#6517=CARTESIAN_POINT ( 'NONE',  ( -65.47859922179033276, 0.5000000000000490719, -11.38422848940298593 ) ) ;
#6528=ORIENTED_EDGE ( 'NONE', *, *, #13280, .F. ) ;
#6530=TOROIDAL_SURFACE ( 'NONE', #10262, 9.499999999999998224, 0.5000000000000000000 ) ;
#6536=EDGE_LOOP ( 'NONE', ( #22686, #4258, #17009, #5635 ) ) ;
#6537=ORIENTED_EDGE ( 'NONE', *, *, #13870, .T. ) ;
#6540=DIRECTION ( 'NONE',  ( -1.550910762415566494E-16, -1.000000000000000000, 8.135128085091684243E-31 ) ) ;
#6546=CIRCLE ( 'NONE', #20833, 0.5000000000000029976 ) ;
#6548=CIRCLE ( 'NONE', #8793, 0.5000000000000028866 ) ;
#6549=DIRECTION ( 'NONE',  ( 6.938893903907255199E-15, 1.000000000000000000, 1.158639454543361089E-30 ) ) ;
#6550=EDGE_CURVE ( 'NONE', #18197, #22258, #8405, .T. ) ;
#6554=FACE_OUTER_BOUND ( 'NONE', #17457, .T. ) ;
#6566=VECTOR ( 'NONE', #12938, 1000.000000000000114 ) ;
#6567=ORIENTED_EDGE ( 'NONE', *, *, #11402, .T. ) ;
#6583=AXIS2_PLACEMENT_3D ( 'NONE', #751, #7916, #15074 ) ;
#6584=CARTESIAN_POINT ( 'NONE',  ( -56.87767137932630845, 1.040834085586084257E-13, 8.833333333333415638 ) ) ;
#6589=EDGE_LOOP ( 'NONE', ( #6035, #10167, #20949, #22027 ) ) ;
#6590=ORIENTED_EDGE ( 'NONE', *, *, #17260, .T. ) ;
#6592=CYLINDRICAL_SURFACE ( 'NONE', #15894, 2.550000000000010481 ) ;
#6594=LINE ( 'NONE', #13768, #10867 ) ;
#6595=ORIENTED_EDGE ( 'NONE', *, *, #1471, .T. ) ;
#6596=DIRECTION ( 'NONE',  ( 1.000000000000000000, 2.220446049250313081E-16, -3.656342123407104498E-48 ) ) ;
#6597=LINE ( 'NONE', #19290, #21395 ) ;
#6600=CYLINDRICAL_SURFACE ( 'NONE', #3928, 4.000000000000023981 ) ;
#6603=CARTESIAN_POINT ( 'NONE',  ( -89.70000000000057128, -6.245004513516505540E-14, -2.000000000000001776 ) ) ;
#6609=ORIENTED_EDGE ( 'NONE', *, *, #3375, .F. ) ;
#6612=ORIENTED_EDGE ( 'NONE', *, *, #11577, .T. ) ;
#6614=VERTEX_POINT ( 'NONE', #16482 ) ;
#6619=CARTESIAN_POINT ( 'NONE',  ( -64.00000000000045475, 3.200000000000057021, -1.999999999999974021 ) ) ;
#6636=EDGE_LOOP ( 'NONE', ( #2061, #14459, #4024, #14560 ) ) ;
#6649=EDGE_LOOP ( 'NONE', ( #1831, #17391, #8146, #10883 ) ) ;
#6650=CARTESIAN_POINT ( 'NONE',  ( -66.55000000000046612, 3.200000000000056577, -1.999999999999974021 ) ) ;
#6654=FACE_OUTER_BOUND ( 'NONE', #6669, .T. ) ;
#6660=TOROIDAL_SURFACE ( 'NONE', #6301, 4.500000000000002665, 0.5000000000000000000 ) ;
#6662=EDGE_CURVE ( 'NONE', #278, #23028, #6690, .T. ) ;
#6669=EDGE_LOOP ( 'NONE', ( #6038, #16378, #6696, #10030 ) ) ;
#6673=ORIENTED_EDGE ( 'NONE', *, *, #15570, .F. ) ;
#6675=CYLINDRICAL_SURFACE ( 'NONE', #8035, 0.5000000000000016653 ) ;
#6677=ORIENTED_EDGE ( 'NONE', *, *, #8005, .F. ) ;
#6679=AXIS2_PLACEMENT_3D ( 'NONE', #18686, #2573, #9758 ) ;
#6686=AXIS2_PLACEMENT_3D ( 'NONE', #23188, #12339, #1533 ) ;
#6690=CIRCLE ( 'NONE', #7068, 2.550000000000010481 ) ;
#6691=DIRECTION ( 'NONE',  ( -2.220446049250313081E-16, 1.000000000000000000, -7.025792437124636392E-31 ) ) ;
#6692=CARTESIAN_POINT ( 'NONE',  ( -42.54314575050799618, 5.299999999999998934, 8.000000000000035527 ) ) ;
#6696=ORIENTED_EDGE ( 'NONE', *, *, #15570, .T. ) ;
#6697=ORIENTED_EDGE ( 'NONE', *, *, #6289, .T. ) ;
#6700=VECTOR ( 'NONE', #2961, 1000.000000000000000 ) ;
#6706=CARTESIAN_POINT ( 'NONE',  ( -55.05572809000126711, 3.200000000000022382, -7.500000000000034639 ) ) ;
#6712=FACE_OUTER_BOUND ( 'NONE', #19626, .T. ) ;
#6713=CARTESIAN_POINT ( 'NONE',  ( -95.70000000000071338, 0.5000000000000073275, 1.000000000000070166 ) ) ;
#6715=DIRECTION ( 'NONE',  ( 1.281898970984144184E-30, 1.000000000000000000, 6.938893903907263876E-15 ) ) ;
#6717=FACE_OUTER_BOUND ( 'NONE', #18842, .T. ) ;
#6718=CYLINDRICAL_SURFACE ( 'NONE', #9504, 0.5000000000000016653 ) ;
#6719=CIRCLE ( 'NONE', #5604, 6.000000000000036415 ) ;
#6720=DIRECTION ( 'NONE',  ( -1.000000000000000000, 1.550910762415502399E-16, 0.000000000000000000 ) ) ;
#6723=CYLINDRICAL_SURFACE ( 'NONE', #2943, 2.550000000000010481 ) ;
#6746=CARTESIAN_POINT ( 'NONE',  ( -42.54314575050796776, 7.499999999999992895, -8.000000000000035527 ) ) ;
#6754=EDGE_LOOP ( 'NONE', ( #14079, #6088, #8173, #9163 ) ) ;
#6756=VECTOR ( 'NONE', #2279, 1000.000000000000000 ) ;
#6757=EDGE_LOOP ( 'NONE', ( #7768, #6016, #20333, #4861 ) ) ;
#6763=CARTESIAN_POINT ( 'NONE',  ( -47.82842712474658242, 4.371572875253824542, -7.500000000000007105 ) ) ;
#6766=FACE_OUTER_BOUND ( 'NONE', #1101, .T. ) ;
#6772=DIRECTION ( 'NONE',  ( -1.000000000000000000, 1.700709290173333260E-16, 0.000000000000000000 ) ) ;
#6783=EDGE_CURVE ( 'NONE', #10966, #19955, #15061, .T. ) ;
#6790=CARTESIAN_POINT ( 'NONE',  ( -6.746326818733313857, 0.5000000000001045830, 27.22340457528590818 ) ) ;
#6798=DIRECTION ( 'NONE',  ( 1.000000000000000000, 2.220446049250313081E-16, -3.656342123407315983E-48 ) ) ;
#6803=DIRECTION ( 'NONE',  ( -1.000000000000000000, 1.550910762415496482E-16, -6.938893903907184004E-16 ) ) ;
#6813=ORIENTED_EDGE ( 'NONE', *, *, #18447, .F. ) ;
#6814=ADVANCED_FACE ( 'NONE', ( #13083 ), #22088, .T. ) ;
#6815=VERTEX_POINT ( 'NONE', #2603 ) ;
#6818=ORIENTED_EDGE ( 'NONE', *, *, #11577, .F. ) ;
#6825=VERTEX_POINT ( 'NONE', #4017 ) ;
#6827=TOROIDAL_SURFACE ( 'NONE', #22987, 3.299999999999999822, 0.5000000000000000000 ) ;
#6837=CARTESIAN_POINT ( 'NONE',  ( -50.65685424949274562, -0.5000000000001045830, 8.000000000000062172 ) ) ;
#6844=ORIENTED_EDGE ( 'NONE', *, *, #10877, .F. ) ;
#6847=DIRECTION ( 'NONE',  ( 0.000000000000000000, 0.000000000000000000, 1.000000000000000000 ) ) ;
#6856=DIRECTION ( 'NONE',  ( 1.550910762415566494E-16, 1.000000000000000000, -8.135128085091684243E-31 ) ) ;
#6857=CARTESIAN_POINT ( 'NONE',  ( -95.20000000000061391, -0.5000000000000975886, 1.000000000000028644 ) ) ;
#6858=CIRCLE ( 'NONE', #14762, 4.000000000000023981 ) ;
#6860=VECTOR ( 'NONE', #21272, 1000.000000000000000 ) ;
#6862=ADVANCED_FACE ( 'NONE', ( #15300 ), #6723, .F. ) ;
#6864=CIRCLE ( 'NONE', #1980, 0.5000000000000028866 ) ;
#6867=CARTESIAN_POINT ( 'NONE',  ( -64.00000000000045475, 2.700000000000056577, -1.999999999999974021 ) ) ;
#6870=EDGE_CURVE ( 'NONE', #5817, #13979, #16817, .T. ) ;
#6874=VERTEX_POINT ( 'NONE', #6837 ) ;
#6875=ORIENTED_EDGE ( 'NONE', *, *, #183, .F. ) ;
#6876=ORIENTED_EDGE ( 'NONE', *, *, #4360, .T. ) ;
#6878=AXIS2_PLACEMENT_3D ( 'NONE', #18829, #21070, #4471 ) ;
#6879=VERTEX_POINT ( 'NONE', #22493 ) ;
#6886=ORIENTED_EDGE ( 'NONE', *, *, #13870, .F. ) ;
#6887=DIRECTION ( 'NONE',  ( 1.000000000000000000, 2.220446049250300755E-16, 2.081668171172155103E-15 ) ) ;
#6890=DIRECTION ( 'NONE',  ( -1.000000000000000000, 0.000000000000000000, 0.000000000000000000 ) ) ;
#6894=PLANE ( 'NONE',  #3436 ) ;
#6895=CARTESIAN_POINT ( 'NONE',  ( -45.56568542494948559, -2.108831175456959972, 8.000000000000062172 ) ) ;
#6899=AXIS2_PLACEMENT_3D ( 'NONE', #16733, #16848, #18627 ) ;
#6903=AXIS2_PLACEMENT_3D ( 'NONE', #2119, #21893, #9306 ) ;
#6906=DIRECTION ( 'NONE',  ( -1.000000000000000000, 1.577021341797084002E-16, -9.777532319141921008E-15 ) ) ;
#6908=EDGE_LOOP ( 'NONE', ( #5613, #20840, #4979, #16176 ) ) ;
#6914=CARTESIAN_POINT ( 'NONE',  ( -50.65685424949267457, 7.200000000000018829, -7.500000000000034639 ) ) ;
#6916=AXIS2_PLACEMENT_3D ( 'NONE', #6320, #13494, #8435 ) ;
#6922=CARTESIAN_POINT ( 'NONE',  ( -45.37157287525403149, -6.828427124746218269, -7.500000000000034639 ) ) ;
#6927=CYLINDRICAL_SURFACE ( 'NONE', #20130, 10.00000000000006395 ) ;
#6929=DIRECTION ( 'NONE',  ( -1.000000000000000000, 1.517883041479696593E-16, 0.000000000000000000 ) ) ;
#6942=EDGE_CURVE ( 'NONE', #10886, #19955, #22102, .T. ) ;
#6948=DIRECTION ( 'NONE',  ( 1.000000000000000000, -1.424116703980815236E-16, -2.931272055834072749E-32 ) ) ;
#6951=EDGE_CURVE ( 'NONE', #6327, #1919, #1320, .T. ) ;
#6956=CARTESIAN_POINT ( 'NONE',  ( -55.25320565519140104, -3.200000000000108979, 7.500000000000047962 ) ) ;
#6961=CARTESIAN_POINT ( 'NONE',  ( -42.54314575050795355, 4.799999999999991829, -7.500000000000007105 ) ) ;
#6964=CARTESIAN_POINT ( 'NONE',  ( -95.70000000000065654, -0.5000000000000975886, -2.000000000000029310 ) ) ;
#6968=ADVANCED_FACE ( 'NONE', ( #10357, #21202, #12225 ), #17528, .T. ) ;
#6972=ADVANCED_FACE ( 'NONE', ( #3873 ), #14590, .F. ) ;
#6982=CARTESIAN_POINT ( 'NONE',  ( -50.65685424949275983, -3.200000000000108979, -8.000000000000007105 ) ) ;
#6983=DIRECTION ( 'NONE',  ( -1.000000000000000000, 0.000000000000000000, 0.000000000000000000 ) ) ;
#6987=CARTESIAN_POINT ( 'NONE',  ( -90.63385214007837476, -2.700000000000084110, -7.926881151201908615 ) ) ;
#6990=DIRECTION ( 'NONE',  ( -2.013525853228507892E-32, -6.902532920683810383E-31, 1.000000000000000000 ) ) ;
#6997=DIRECTION ( 'NONE',  ( -1.550910762415566494E-16, -1.000000000000000000, 8.135128085091684243E-31 ) ) ;
#6998=VERTEX_POINT ( 'NONE', #14249 ) ;
#7004=EDGE_LOOP ( 'NONE', ( #9825, #5078, #12505, #1454 ) ) ;
#7005=EDGE_LOOP ( 'NONE', ( #12511, #9190, #3946, #11205 ) ) ;
#7014=DIRECTION ( 'NONE',  ( -1.000000000000000000, 1.550910762415566494E-16, -8.566929763922626680E-48 ) ) ;
#7020=DIRECTION ( 'NONE',  ( 1.000000000000000000, 2.168404344970995063E-16, 0.000000000000000000 ) ) ;
#7024=VERTEX_POINT ( 'NONE', #10590 ) ;
#7025=AXIS2_PLACEMENT_3D ( 'NONE', #9687, #756, #20395 ) ;
#7037=DIRECTION ( 'NONE',  ( -1.000000000000000000, 1.734723475976796001E-16, 0.000000000000000000 ) ) ;
#7053=AXIS2_PLACEMENT_3D ( 'NONE', #15843, #16190, #17738 ) ;
#7054=CARTESIAN_POINT ( 'NONE',  ( -45.91923881554285458, 2.462384566050197954, -8.000000000000007105 ) ) ;
#7059=CIRCLE ( 'NONE', #2523, 5.500000000000046185 ) ;
#7061=ORIENTED_EDGE ( 'NONE', *, *, #1321, .F. ) ;
#7068=AXIS2_PLACEMENT_3D ( 'NONE', #18152, #9210, #16021 ) ;
#7078=FACE_OUTER_BOUND ( 'NONE', #15224, .T. ) ;
#7079=AXIS2_PLACEMENT_3D ( 'NONE', #4886, #19618, #16075 ) ;
#7080=CARTESIAN_POINT ( 'NONE',  ( -43.46238456605044576, 4.919238815542535725, 7.500000000000034639 ) ) ;
#7084=EDGE_CURVE ( 'NONE', #2832, #4603, #11054, .T. ) ;
#7088=EDGE_LOOP ( 'NONE', ( #18124, #22235, #5463, #12748 ) ) ;
#7091=VECTOR ( 'NONE', #18834, 1000.000000000000000 ) ;
#7092=EDGE_CURVE ( 'NONE', #20537, #4165, #2565, .T. ) ;
#7093=ORIENTED_EDGE ( 'NONE', *, *, #14288, .F. ) ;
#7103=ORIENTED_EDGE ( 'NONE', *, *, #653, .T. ) ;
#7105=CARTESIAN_POINT ( 'NONE',  ( -50.65685424949263904, -7.200000000000071232, -7.500000000000034639 ) ) ;
#7110=DIRECTION ( 'NONE',  ( -1.000000000000000000, 1.700709290173333260E-16, 0.000000000000000000 ) ) ;
#7111=DIRECTION ( 'NONE',  ( -0.8122328620674192923, 0.000000000000000000, -0.5833333333333257098 ) ) ;
#7124=EDGE_CURVE ( 'NONE', #15019, #1880, #16792, .T. ) ;
#7126=AXIS2_PLACEMENT_3D ( 'NONE', #14308, #10426, #23017 ) ;
#7127=VERTEX_POINT ( 'NONE', #16685 ) ;
#7129=AXIS2_PLACEMENT_3D ( 'NONE', #5364, #12407, #10419 ) ;
#7133=CARTESIAN_POINT ( 'NONE',  ( -0.5000000000000420775, 1.999999999999932498, -8.000000000000035527 ) ) ;
#7141=CARTESIAN_POINT ( 'NONE',  ( -91.14322581977724269, -1.179611963664228824E-13, 6.823838874241872077 ) ) ;
#7144=DIRECTION ( 'NONE',  ( -0.7071067811865233699, 0.7071067811865715536, 0.000000000000000000 ) ) ;
#7150=ORIENTED_EDGE ( 'NONE', *, *, #10075, .T. ) ;
#7155=LINE ( 'NONE', #17608, #156 ) ;
#7158=DIRECTION ( 'NONE',  ( 0.7071067811865491270, 0.7071067811865461294, 1.565905175853767167E-16 ) ) ;
#7160=CYLINDRICAL_SURFACE ( 'NONE', #22859, 2.000000000000015543 ) ;
#7161=VECTOR ( 'NONE', #7699, 1000.000000000000000 ) ;
#7167=DIRECTION ( 'NONE',  ( 1.000000000000000000, 1.479114197289388027E-30, -2.013525853228518840E-32 ) ) ;
#7168=EDGE_CURVE ( 'NONE', #22149, #10662, #17576, .T. ) ;
#7178=DIRECTION ( 'NONE',  ( -1.000000000000000000, 1.550910762415526064E-16, 0.000000000000000000 ) ) ;
#7187=DIRECTION ( 'NONE',  ( -0.9878135252003119593, -2.699958717473711339E-16, 0.1556420233463085001 ) ) ;
#7193=( NAMED_UNIT ( * ) SI_UNIT ( $, .STERADIAN. ) SOLID_ANGLE_UNIT ( ) );
#7200=ORIENTED_EDGE ( 'NONE', *, *, #336, .T. ) ;
#7208=PLANE ( 'NONE',  #15237 ) ;
#7213=DIRECTION ( 'NONE',  ( 0.7071067811865464625, 0.7071067811865486830, 2.121016688166348642E-16 ) ) ;
#7216=EDGE_CURVE ( 'NONE', #22937, #20537, #18815, .T. ) ;
#7219=AXIS2_PLACEMENT_3D ( 'NONE', #19015, #17232, #15809 ) ;
#7222=FACE_OUTER_BOUND ( 'NONE', #19805, .T. ) ;
#7225=ORIENTED_EDGE ( 'NONE', *, *, #9053, .F. ) ;
#7227=ADVANCED_FACE ( 'NONE', ( #10110 ), #21052, .T. ) ;
#7236=FACE_OUTER_BOUND ( 'NONE', #20967, .T. ) ;
#7248=CARTESIAN_POINT ( 'NONE',  ( -67.28510754798018922, 0.5000000000000143219, 12.22107821754958579 ) ) ;
#7253=PLANE ( 'NONE',  #7126 ) ;
#7269=CIRCLE ( 'NONE', #20429, 10.00000000000006395 ) ;
#7273=CARTESIAN_POINT ( 'NONE',  ( -89.70000000000064233, 0.5000000000000490719, -2.000000000000001776 ) ) ;
#7276=CIRCLE ( 'NONE', #4637, 6.000000000000037303 ) ;
#7282=DIRECTION ( 'NONE',  ( -0.9706398123736329486, 1.505375731439247187E-16, -0.2405376366294442458 ) ) ;
#7285=DIRECTION ( 'NONE',  ( -1.000000000000000000, 1.550910762415566494E-16, -8.566929763922626680E-48 ) ) ;
#7291=AXIS2_PLACEMENT_3D ( 'NONE', #11161, #16551, #5876 ) ;
#7295=ORIENTED_EDGE ( 'NONE', *, *, #15709, .F. ) ;
#7299=DIRECTION ( 'NONE',  ( 1.000000000000000000, 1.144237745222090235E-17, -1.939787525279694125E-32 ) ) ;
#7300=ORIENTED_EDGE ( 'NONE', *, *, #10778, .T. ) ;
#7302=DIRECTION ( 'NONE',  ( -1.000000000000000000, 6.640738306473671271E-15, 4.480856046118915636E-31 ) ) ;
#7306=CARTESIAN_POINT ( 'NONE',  ( -55.25320565519140104, -2.700000000000049472, 10.00000000000007816 ) ) ;
#7307=FACE_OUTER_BOUND ( 'NONE', #18534, .T. ) ;
#7310=FACE_OUTER_BOUND ( 'NONE', #13093, .T. ) ;
#7311=AXIS2_PLACEMENT_3D ( 'NONE', #12989, #20164, #21819 ) ;
#7317=ORIENTED_EDGE ( 'NONE', *, *, #12256, .F. ) ;
#7322=AXIS2_PLACEMENT_3D ( 'NONE', #11438, #2502, #13450 ) ;
#7327=DIRECTION ( 'NONE',  ( 2.220446049250313081E-16, -1.000000000000000000, 7.025792437124636392E-31 ) ) ;
#7334=CIRCLE ( 'NONE', #201, 0.8000000000000090372 ) ;
#7335=AXIS2_PLACEMENT_3D ( 'NONE', #21219, #8497, #19548 ) ;
#7337=CARTESIAN_POINT ( 'NONE',  ( -67.28510754798023186, 3.200000000000022382, 12.22107821754961421 ) ) ;
#7344=ORIENTED_EDGE ( 'NONE', *, *, #6662, .F. ) ;
#7348=CYLINDRICAL_SURFACE ( 'NONE', #12095, 4.000000000000023981 ) ;
#7353=CYLINDRICAL_SURFACE ( 'NONE', #755, 10.00000000000006395 ) ;
#7356=DIRECTION ( 'NONE',  ( 1.000000000000000000, -1.424116703980815236E-16, -2.931272055834072749E-32 ) ) ;
#7375=ORIENTED_EDGE ( 'NONE', *, *, #20908, .T. ) ;
#7379=PLANE ( 'NONE',  #18108 ) ;
#7382=ADVANCED_FACE ( 'NONE', ( #1853 ), #5607, .T. ) ;
#7391=CARTESIAN_POINT ( 'NONE',  ( -95.20000000000067075, 0.5000000000000073275, -1.999999999999974021 ) ) ;
#7397=CARTESIAN_POINT ( 'NONE',  ( -3.336453936897160411, -2.700000000000098321, -21.17547853860576978 ) ) ;
#7404=VECTOR ( 'NONE', #22936, 1000.000000000000000 ) ;
#7410=CARTESIAN_POINT ( 'NONE',  ( -42.54314575050785407, -8.000000000000021316, 8.000000000000007105 ) ) ;
#7418=AXIS2_PLACEMENT_3D ( 'NONE', #2456, #13172, #18811 ) ;
#7419=EDGE_CURVE ( 'NONE', #6879, #17750, #11218, .T. ) ;
#7426=VECTOR ( 'NONE', #19443, 1000.000000000000000 ) ;
#7446=DIRECTION ( 'NONE',  ( -0.2405376366294442736, 3.887513393996810040E-17, 0.9706398123736330597 ) ) ;
#7453=ORIENTED_EDGE ( 'NONE', *, *, #14993, .F. ) ;
#7454=ORIENTED_EDGE ( 'NONE', *, *, #7975, .T. ) ;
#7462=ORIENTED_EDGE ( 'NONE', *, *, #17174, .T. ) ;
#7467=DIRECTION ( 'NONE',  ( 0.000000000000000000, 0.000000000000000000, 1.000000000000000000 ) ) ;
#7471=CYLINDRICAL_SURFACE ( 'NONE', #13257, 0.5000000000000037748 ) ;
#7473=DIRECTION ( 'NONE',  ( 2.013525853228507892E-32, 6.902532920683810383E-31, -1.000000000000000000 ) ) ;
#7478=VECTOR ( 'NONE', #9264, 1000.000000000000000 ) ;
#7479=CARTESIAN_POINT ( 'NONE',  ( -65.00000000000052580, 2.700000000000063238, 3.000000000000002665 ) ) ;
#7485=VERTEX_POINT ( 'NONE', #7054 ) ;
#7486=ORIENTED_EDGE ( 'NONE', *, *, #2803, .F. ) ;
#7487=ADVANCED_FACE ( 'NONE', ( #21523 ), #23262, .T. ) ;
#7493=DIRECTION ( 'NONE',  ( -2.013525853228507892E-32, -6.902532920683810383E-31, 1.000000000000000000 ) ) ;
#7495=CARTESIAN_POINT ( 'NONE',  ( -50.65685424949267457, 7.200000000000018829, -7.500000000000034639 ) ) ;
#7496=CYLINDRICAL_SURFACE ( 'NONE', #9258, 6.000000000000047073 ) ;
#7499=ADVANCED_FACE ( 'NONE', ( #11480 ), #12791, .T. ) ;
#7503=FACE_OUTER_BOUND ( 'NONE', #4364, .T. ) ;
#7505=ADVANCED_FACE ( 'NONE', ( #16536 ), #684, .T. ) ;
#7516=CARTESIAN_POINT ( 'NONE',  ( -0.5000000000000559552, -2.000000000000029310, 8.000000000000062172 ) ) ;
#7517=CARTESIAN_POINT ( 'NONE',  ( -55.05572809000118184, -2.700000000000125855, -8.000000000000062172 ) ) ;
#7522=CARTESIAN_POINT ( 'NONE',  ( -6.000000000000116351, -7.500000000000027534, -8.000000000000007105 ) ) ;
#7544=CARTESIAN_POINT ( 'NONE',  ( -47.82842712474641189, -4.371572875253856516, 7.500000000000047962 ) ) ;
#7548=EDGE_CURVE ( 'NONE', #2913, #14457, #11143, .T. ) ;
#7549=CARTESIAN_POINT ( 'NONE',  ( -43.10883117545719045, 7.499999999999992895, 7.500000000000007105 ) ) ;
#7551=DIRECTION ( 'NONE',  ( 1.000000000000000000, 2.220446049250314067E-16, -5.825996348268307008E-33 ) ) ;
#7558=FACE_OUTER_BOUND ( 'NONE', #21590, .T. ) ;
#7563=CIRCLE ( 'NONE', #20343, 4.000000000000023981 ) ;
#7565=ORIENTED_EDGE ( 'NONE', *, *, #2207, .T. ) ;
#7566=ORIENTED_EDGE ( 'NONE', *, *, #5746, .T. ) ;
#7571=ORIENTED_EDGE ( 'NONE', *, *, #13581, .F. ) ;
#7574=VERTEX_POINT ( 'NONE', #2315 ) ;
#7578=ADVANCED_FACE ( 'NONE', ( #18436 ), #9495, .T. ) ;
#7582=DIRECTION ( 'NONE',  ( -0.7071067811865491270, -0.7071067811865461294, -1.565905175853767167E-16 ) ) ;
#7585=DIRECTION ( 'NONE',  ( 2.013525853228507892E-32, 6.902532920683810383E-31, -1.000000000000000000 ) ) ;
#7608=DIRECTION ( 'NONE',  ( -1.000000000000000000, -2.220446049250301001E-16, 0.000000000000000000 ) ) ;
#7618=FILL_AREA_STYLE ('',( #13150 ) ) ;
#7622=VERTEX_POINT ( 'NONE', #8314 ) ;
#7626=VERTEX_POINT ( 'NONE', #10186 ) ;
#7628=VECTOR ( 'NONE', #1557, 1000.000000000000000 ) ;
#7634=CYLINDRICAL_SURFACE ( 'NONE', #6023, 6.000000000000047073 ) ;
#7635=CARTESIAN_POINT ( 'NONE',  ( -3.336453936897187944, 0.5000000000000628386, -21.17547853860574136 ) ) ;
#7640=DIRECTION ( 'NONE',  ( -1.815210279346896549E-30, 6.902532920684321857E-31, -1.000000000000000000 ) ) ;
#7641=DIRECTION ( 'NONE',  ( -2.013525853228518840E-32, 6.902532920683810383E-31, -1.000000000000000000 ) ) ;
#7647=AXIS2_PLACEMENT_3D ( 'NONE', #22747, #8400, #21228 ) ;
#7650=AXIS2_PLACEMENT_3D ( 'NONE', #8729, #8499, #6983 ) ;
#7655=ORIENTED_EDGE ( 'NONE', *, *, #3221, .T. ) ;
#7657=DIRECTION ( 'NONE',  ( -1.000000000000000000, -1.110223024625164429E-16, -2.013525853228515555E-32 ) ) ;
#7669=DIRECTION ( 'NONE',  ( 0.7071067811865485719, -0.7071067811865463515, -1.010793663541191485E-16 ) ) ;
#7674=FACE_OUTER_BOUND ( 'NONE', #5405, .T. ) ;
#7677=DIRECTION ( 'NONE',  ( 2.013525853228507892E-32, 6.902532920683810383E-31, -1.000000000000000000 ) ) ;
#7684=VERTEX_POINT ( 'NONE', #22433 ) ;
#7689=VERTEX_POINT ( 'NONE', #19240 ) ;
#7697=CARTESIAN_POINT ( 'NONE',  ( -6.000000000000088818, -2.000000000000050182, -17.72029585817572084 ) ) ;
#7699=DIRECTION ( 'NONE',  ( -1.550910762415566494E-16, -1.000000000000000000, 8.135128085091684243E-31 ) ) ;
#7700=LINE ( 'NONE', #18285, #19258 ) ;
#7708=DIRECTION ( 'NONE',  ( 1.000000000000000000, 2.220446049250313081E-16, 4.712618736834399899E-47 ) ) ;
#7711=ADVANCED_FACE ( 'NONE', ( #3601 ), #7253, .T. ) ;
#7715=EDGE_LOOP ( 'NONE', ( #13706, #16061, #17246, #4033 ) ) ;
#7718=CARTESIAN_POINT ( 'NONE',  ( -42.54314575050795355, 3.999999999999996447, -7.500000000000007105 ) ) ;
#7730=FACE_BOUND ( 'NONE', #8941, .T. ) ;
#7736=ORIENTED_EDGE ( 'NONE', *, *, #3866, .F. ) ;
#7737=CARTESIAN_POINT ( 'NONE',  ( -87.15000000000065938, 3.200000000000057465, -2.000000000000001332 ) ) ;
#7741=DIRECTION ( 'NONE',  ( 2.013525853228518840E-32, -6.902532920683810383E-31, 1.000000000000000000 ) ) ;
#7748=EDGE_LOOP ( 'NONE', ( #23241, #2613, #18390, #10774 ) ) ;
#7749=FACE_OUTER_BOUND ( 'NONE', #16800, .T. ) ;
#7754=DIRECTION ( 'NONE',  ( -1.000000000000000000, -1.734723475976799009E-15, -9.165585228034679171E-32 ) ) ;
#7755=CARTESIAN_POINT ( 'NONE',  ( -45.01801948466079040, -6.474873734152946092, 8.000000000000021316 ) ) ;
#7760=ORIENTED_EDGE ( 'NONE', *, *, #3171, .T. ) ;
#7768=ORIENTED_EDGE ( 'NONE', *, *, #14555, .T. ) ;
#7788=ADVANCED_FACE ( 'NONE', ( #10880 ), #11595, .T. ) ;
#7795=EDGE_LOOP ( 'NONE', ( #11989, #14879, #8875, #7565 ) ) ;
#7797=ORIENTED_EDGE ( 'NONE', *, *, #2396, .T. ) ;
#7798=AXIS2_PLACEMENT_3D ( 'NONE', #9634, #7754, #21877 ) ;
#7808=DIRECTION ( 'NONE',  ( 1.000000000000000000, 1.479114197289387852E-30, -2.013525853228518840E-32 ) ) ;
#7809=CIRCLE ( 'NONE', #20576, 2.550000000000010481 ) ;
#7811=CARTESIAN_POINT ( 'NONE',  ( -55.25320565519150051, 2.700000000000098321, 7.500000000000062172 ) ) ;
#7818=VECTOR ( 'NONE', #3681, 1000.000000000000000 ) ;
#7823=AXIS2_PLACEMENT_3D ( 'NONE', #14277, #17675, #12025 ) ;
#7826=ORIENTED_EDGE ( 'NONE', *, *, #3551, .F. ) ;
#7829=AXIS2_PLACEMENT_3D ( 'NONE', #1424, #8599, #15763 ) ;
#7835=ORIENTED_EDGE ( 'NONE', *, *, #15896, .F. ) ;
#7838=CARTESIAN_POINT ( 'NONE',  ( -42.54314575050785407, -4.000000000000034639, -7.500000000000007105 ) ) ;
#7850=( LENGTH_UNIT ( ) NAMED_UNIT ( * ) SI_UNIT ( .MILLI., .METRE. ) );
#7855=VERTEX_POINT ( 'NONE', #305 ) ;
#7858=FACE_BOUND ( 'NONE', #11465, .T. ) ;
#7862=FACE_OUTER_BOUND ( 'NONE', #8476, .T. ) ;
#7864=DIRECTION ( 'NONE',  ( 0.000000000000000000, -1.000000000000000000, 0.000000000000000000 ) ) ;
#7877=EDGE_LOOP ( 'NONE', ( #13482, #18054, #21727, #13445 ) ) ;
#7883=ADVANCED_FACE ( 'NONE', ( #1936 ), #12349, .T. ) ;
#7907=ORIENTED_EDGE ( 'NONE', *, *, #20591, .T. ) ;
#7908=UNCERTAINTY_MEASURE_WITH_UNIT (LENGTH_MEASURE( 1.000000000000000082E-05 ), #7850, 'distance_accuracy_value', 'NONE');
#7916=DIRECTION ( 'NONE',  ( -0.7071067811865485719, 0.7071067811865464625, 1.010793663541191362E-16 ) ) ;
#7919=ADVANCED_FACE ( 'NONE', ( #20068 ), #13871, .T. ) ;
#7922=DIRECTION ( 'NONE',  ( 1.000000000000000000, 2.220446049250307657E-16, 0.000000000000000000 ) ) ;
#7945=ADVANCED_FACE ( 'NONE', ( #22061 ), #8598, .T. ) ;
#7959=EDGE_CURVE ( 'NONE', #9134, #3579, #14608, .T. ) ;
#7965=VECTOR ( 'NONE', #21273, 1000.000000000000114 ) ;
#7966=ORIENTED_EDGE ( 'NONE', *, *, #13293, .T. ) ;
#7975=EDGE_CURVE ( 'NONE', #4281, #15019, #13505, .T. ) ;
#7990=DIRECTION ( 'NONE',  ( -2.220446049250313081E-16, 1.000000000000000000, -7.025792437124636392E-31 ) ) ;
#8005=EDGE_CURVE ( 'NONE', #22532, #2832, #16489, .T. ) ;
#8013=CARTESIAN_POINT ( 'NONE',  ( -3.200000000000119194, 1.999999999999911626, 7.500000000000062172 ) ) ;
#8014=AXIS2_PLACEMENT_3D ( 'NONE', #10107, #9874, #4694 ) ;
#8015=DIRECTION ( 'NONE',  ( 1.000000000000000000, 1.156482317317863245E-14, 0.000000000000000000 ) ) ;
#8018=AXIS2_PLACEMENT_3D ( 'NONE', #3418, #14469, #21653 ) ;
#8023=DIRECTION ( 'NONE',  ( -1.000000000000000000, -1.908195823574478022E-14, 2.087219286295281359E-14 ) ) ;
#8030=ORIENTED_EDGE ( 'NONE', *, *, #15423, .F. ) ;
#8033=AXIS2_PLACEMENT_3D ( 'NONE', #17137, #13511, #937 ) ;
#8035=AXIS2_PLACEMENT_3D ( 'NONE', #6790, #16177, #19252 ) ;
#8043=DIRECTION ( 'NONE',  ( 2.013525853228518840E-32, -6.902532920683810383E-31, 1.000000000000000000 ) ) ;
#8061=ORIENTED_EDGE ( 'NONE', *, *, #19283, .T. ) ;
#8064=DIRECTION ( 'NONE',  ( 0.5833333333333320381, 1.429810390713075314E-30, -0.8122328620674146293 ) ) ;
#8070=DIRECTION ( 'NONE',  ( -0.2405376366294442736, -2.775557561562981331E-17, 0.9706398123736330597 ) ) ;
#8074=FACE_BOUND ( 'NONE', #4758, .T. ) ;
#8076=CARTESIAN_POINT ( 'NONE',  ( -55.05572809000130974, 1.387778780781445676E-14, -8.000000000000035527 ) ) ;
#8082=CARTESIAN_POINT ( 'NONE',  ( -91.02295700146254376, -1.040834085586084257E-13, 6.338518968055040226 ) ) ;
#8087=VERTEX_POINT ( 'NONE', #7737 ) ;
#8098=VERTEX_POINT ( 'NONE', #11032 ) ;
#8099=CIRCLE ( 'NONE', #3588, 0.5000000000000029976 ) ;
#8104=DIRECTION ( 'NONE',  ( -0.7071067811865485719, 0.7071067811865464625, 1.010793663541191485E-16 ) ) ;
#8110=EDGE_CURVE ( 'NONE', #22558, #12086, #14676, .T. ) ;
#8112=EDGE_CURVE ( 'NONE', #10141, #22558, #6124, .T. ) ;
#8122=AXIS2_PLACEMENT_3D ( 'NONE', #1062, #2690, #13639 ) ;
#8123=DIRECTION ( 'NONE',  ( 0.000000000000000000, 0.000000000000000000, 1.000000000000000000 ) ) ;
#8126=CARTESIAN_POINT ( 'NONE',  ( -47.82842712474651137, 4.371572875253824542, 7.500000000000020428 ) ) ;
#8129=CARTESIAN_POINT ( 'NONE',  ( -42.54314575050792513, 3.999999999999996447, 16.42537846091821052 ) ) ;
#8134=ADVANCED_FACE ( 'NONE', ( #16323 ), #3122, .T. ) ;
#8137=DIRECTION ( 'NONE',  ( -1.550910762415566494E-16, -1.000000000000000000, 8.135128085091684243E-31 ) ) ;
#8140=ADVANCED_FACE ( 'NONE', ( #14798 ), #5751, .T. ) ;
#8146=ORIENTED_EDGE ( 'NONE', *, *, #17174, .F. ) ;
#8147=VERTEX_POINT ( 'NONE', #14563 ) ;
#8148=ORIENTED_EDGE ( 'NONE', *, *, #17919, .T. ) ;
#8156=CIRCLE ( 'NONE', #21317, 0.5000000000000019984 ) ;
#8157=CARTESIAN_POINT ( 'NONE',  ( -95.20000000000052864, -2.700000000000119194, 1.000000000000000888 ) ) ;
#8159=LINE ( 'NONE', #22626, #16246 ) ;
#8165=AXIS2_PLACEMENT_3D ( 'NONE', #18755, #14552, #8166 ) ;
#8166=DIRECTION ( 'NONE',  ( 1.000000000000000000, 2.220446049250313081E-16, -3.656342123407104498E-48 ) ) ;
#8167=DIRECTION ( 'NONE',  ( 0.7071067811865485719, -0.7071067811865464625, -1.010793663541191485E-16 ) ) ;
#8173=ORIENTED_EDGE ( 'NONE', *, *, #6360, .T. ) ;
#8174=VERTEX_POINT ( 'NONE', #12797 ) ;
#8176=EDGE_LOOP ( 'NONE', ( #4726, #3825, #8872, #5847 ) ) ;
#8181=ORIENTED_EDGE ( 'NONE', *, *, #11456, .F. ) ;
#8184=DIRECTION ( 'NONE',  ( 1.000000000000000000, 2.220446049250314067E-16, -5.825996348268307008E-33 ) ) ;
#8186=DIRECTION ( 'NONE',  ( -1.000000000000000000, 3.553773787591352645E-14, 0.000000000000000000 ) ) ;
#8200=VERTEX_POINT ( 'NONE', #12683 ) ;
#8202=AXIS2_PLACEMENT_3D ( 'NONE', #21879, #12939, #11169 ) ;
#8207=EDGE_LOOP ( 'NONE', ( #22438, #2936, #18497, #22407 ) ) ;
#8209=MECHANICAL_DESIGN_GEOMETRIC_PRESENTATION_REPRESENTATION('',(#1083),#8968);
#8214=CARTESIAN_POINT ( 'NONE',  ( -67.40537636629493079, 2.700000000000021938, 12.70639812373644517 ) ) ;
#8222=EDGE_CURVE ( 'NONE', #5689, #15196, #2443, .T. ) ;
#8227=LINE ( 'NONE', #6584, #11766 ) ;
#8228=DIRECTION ( 'NONE',  ( 0.1556420233463076119, 0.000000000000000000, 0.9878135252003121813 ) ) ;
#8232=EDGE_CURVE ( 'NONE', #3480, #7127, #3845, .T. ) ;
#8235=CIRCLE ( 'NONE', #14248, 0.5000000000000029976 ) ;
#8236=ORIENTED_EDGE ( 'NONE', *, *, #22926, .T. ) ;
#8241=CARTESIAN_POINT ( 'NONE',  ( -56.54644007500109382, -1.110223024625156540E-13, -8.666666666666655416 ) ) ;
#8244=ORIENTED_EDGE ( 'NONE', *, *, #3392, .F. ) ;
#8255=LINE ( 'NONE', #3199, #20190 ) ;
#8256=CIRCLE ( 'NONE', #13877, 7.200000000000046363 ) ;
#8259=CARTESIAN_POINT ( 'NONE',  ( -61.45000000000044338, 6.301625887772388776E-14, -1.999999999999973577 ) ) ;
#8263=EDGE_CURVE ( 'NONE', #15196, #7689, #6864, .T. ) ;
#8265=ORIENTED_EDGE ( 'NONE', *, *, #20922, .T. ) ;
#8288=CARTESIAN_POINT ( 'NONE',  ( -6.000000000000088818, -5.300000000000027356, -8.000000000000007105 ) ) ;
#8289=DIRECTION ( 'NONE',  ( 0.000000000000000000, -1.000000000000000000, 0.000000000000000000 ) ) ;
#8292=ORIENTED_EDGE ( 'NONE', *, *, #15978, .T. ) ;
#8297=ADVANCED_FACE ( 'NONE', ( #7858, #20567, #4312 ), #4552, .T. ) ;
#8305=DIRECTION ( 'NONE',  ( 2.013525853228507892E-32, 6.902532920683810383E-31, -1.000000000000000000 ) ) ;
#8314=CARTESIAN_POINT ( 'NONE',  ( -65.47859922179033276, 3.200000000000057021, -11.38422848940298593 ) ) ;
#8316=EDGE_LOOP ( 'NONE', ( #22539, #22030, #20274, #2584 ) ) ;
#8318=AXIS2_PLACEMENT_3D ( 'NONE', #5031, #22697, #11860 ) ;
#8326=DIRECTION ( 'NONE',  ( -0.9878135252003126254, -7.334277233329626759E-17, 0.1556420233463035041 ) ) ;
#8335=AXIS2_PLACEMENT_3D ( 'NONE', #16665, #5986, #11149 ) ;
#8339=EDGE_CURVE ( 'NONE', #7626, #21891, #8372, .T. ) ;
#8341=ORIENTED_EDGE ( 'NONE', *, *, #6239, .F. ) ;
#8344=ORIENTED_EDGE ( 'NONE', *, *, #11510, .F. ) ;
#8348=AXIS2_PLACEMENT_3D ( 'NONE', #7838, #9142, #4071 ) ;
#8359=CYLINDRICAL_SURFACE ( 'NONE', #17459, 0.8000000000000090372 ) ;
#8362=CARTESIAN_POINT ( 'NONE',  ( -65.55642023346354108, 0.5000000000000490719, -11.87813525200309783 ) ) ;
#8365=ADVANCED_FACE ( 'NONE', ( #8670 ), #7348, .T. ) ;
#8370=AXIS2_PLACEMENT_3D ( 'NONE', #10983, #73, #9114 ) ;
#8371=ORIENTED_EDGE ( 'NONE', *, *, #4342, .T. ) ;
#8372=CIRCLE ( 'NONE', #17375, 4.500000000000031974 ) ;
#8385=DIRECTION ( 'NONE',  ( 6.938893903907285176E-15, 1.000000000000000000, 2.736361264985384700E-30 ) ) ;
#8387=VECTOR ( 'NONE', #10588, 1000.000000000000000 ) ;
#8388=AXIS2_PLACEMENT_3D ( 'NONE', #18603, #13073, #608 ) ;
#8400=DIRECTION ( 'NONE',  ( -2.220446049250313081E-16, 1.000000000000000000, -7.025792437124636392E-31 ) ) ;
#8405=LINE ( 'NONE', #10046, #7426 ) ;
#8407=ADVANCED_FACE ( 'NONE', ( #19372 ), #21536, .T. ) ;
#8417=CIRCLE ( 'NONE', #6163, 4.000000000000023981 ) ;
#8426=LINE ( 'NONE', #15584, #19633 ) ;
#8435=DIRECTION ( 'NONE',  ( -1.000000000000000000, 0.000000000000000000, 0.000000000000000000 ) ) ;
#8437=LINE ( 'NONE', #18660, #12252 ) ;
#8443=CIRCLE ( 'NONE', #11804, 0.5000000000000004441 ) ;
#8451=FACE_OUTER_BOUND ( 'NONE', #7795, .T. ) ;
#8457=AXIS2_PLACEMENT_3D ( 'NONE', #128, #5065, #21194 ) ;
#8459=AXIS2_PLACEMENT_3D ( 'NONE', #12238, #1781, #14367 ) ;
#8462=CARTESIAN_POINT ( 'NONE',  ( -42.54314575050795355, 3.999999999999996447, -7.500000000000007105 ) ) ;
#8468=CIRCLE ( 'NONE', #8842, 0.5000000000000028866 ) ;
#8472=DIRECTION ( 'NONE',  ( -1.000000000000000000, 1.550910762415526064E-16, 0.000000000000000000 ) ) ;
#8476=EDGE_LOOP ( 'NONE', ( #8181, #17579, #15971, #17534 ) ) ;
#8489=VECTOR ( 'NONE', #11901, 1000.000000000000000 ) ;
#8496=CARTESIAN_POINT ( 'NONE',  ( -9.714451465470119729E-14, -2.775557561562891351E-14, -7.500000000000062172 ) ) ;
#8497=DIRECTION ( 'NONE',  ( -0.6666666666666649643, -4.683861624749726065E-31, -0.7453559924999314523 ) ) ;
#8499=DIRECTION ( 'NONE',  ( 2.013525853228507892E-32, 6.902532920683810383E-31, -1.000000000000000000 ) ) ;
#8518=ORIENTED_EDGE ( 'NONE', *, *, #5746, .F. ) ;
#8526=ORIENTED_EDGE ( 'NONE', *, *, #22790, .T. ) ;
#8531=DIRECTION ( 'NONE',  ( 2.013525853228507892E-32, 6.902532920683810383E-31, -1.000000000000000000 ) ) ;
#8536=LINE ( 'NONE', #4559, #20814 ) ;
#8545=AXIS2_PLACEMENT_3D ( 'NONE', #10904, #16194, #12324 ) ;
#8551=ORIENTED_EDGE ( 'NONE', *, *, #779, .F. ) ;
#8555=ORIENTED_EDGE ( 'NONE', *, *, #8659, .T. ) ;
#8560=AXIS2_PLACEMENT_3D ( 'NONE', #12197, #6691, #19264 ) ;
#8561=CARTESIAN_POINT ( 'NONE',  ( -50.65685424949267457, -7.200000000000049916, 8.000000000000035527 ) ) ;
#8566=FACE_OUTER_BOUND ( 'NONE', #4489, .T. ) ;
#8576=EDGE_LOOP ( 'NONE', ( #21181, #15483, #15541, #18702 ) ) ;
#8577=ORIENTED_EDGE ( 'NONE', *, *, #11696, .T. ) ;
#8591=CARTESIAN_POINT ( 'NONE',  ( -65.55642023346344160, -2.700000000000091216, -11.87813525200317954 ) ) ;
#8598=TOROIDAL_SURFACE ( 'NONE', #1107, 2.500000000000002220, 0.5000000000000000000 ) ;
#8599=DIRECTION ( 'NONE',  ( 2.220446049250314067E-16, -1.000000000000000000, 7.025792437124636392E-31 ) ) ;
#8605=EDGE_LOOP ( 'NONE', ( #22530, #7317, #12616, #15108 ) ) ;
#8607=ORIENTED_EDGE ( 'NONE', *, *, #1810, .F. ) ;
#8610=DIRECTION ( 'NONE',  ( -1.550910762415566494E-16, -1.000000000000000000, 8.135128085091684243E-31 ) ) ;
#8615=CIRCLE ( 'NONE', #1482, 0.4999999999999994449 ) ;
#8617=DIRECTION ( 'NONE',  ( -0.9878135252003127365, 1.532010627492774434E-16, 0.1556420233463029767 ) ) ;
#8620=CARTESIAN_POINT ( 'NONE',  ( -47.47487373415325607, 4.018019484660559471, 7.500000000000007105 ) ) ;
#8635=EDGE_CURVE ( 'NONE', #22909, #17679, #22738, .T. ) ;
#8645=DIRECTION ( 'NONE',  ( 1.550910762415566494E-16, 1.000000000000000000, -8.135128085091684243E-31 ) ) ;
#8659=EDGE_CURVE ( 'NONE', #8098, #17679, #19277, .T. ) ;
#8670=FACE_OUTER_BOUND ( 'NONE', #16868, .T. ) ;
#8671=DIRECTION ( 'NONE',  ( 0.7071067811865490160, 0.7071067811865460184, 1.565905175853766674E-16 ) ) ;
#8676=CARTESIAN_POINT ( 'NONE',  ( -42.54314575050796776, 5.299999999999991829, -8.000000000000035527 ) ) ;
#8683=DIRECTION ( 'NONE',  ( -1.000000000000000000, -1.424116703980846297E-16, 1.095779650622964657E-32 ) ) ;
#8695=EDGE_CURVE ( 'NONE', #18640, #14890, #17426, .T. ) ;
#8696=ORIENTED_EDGE ( 'NONE', *, *, #14993, .T. ) ;
#8699=ORIENTED_EDGE ( 'NONE', *, *, #19579, .F. ) ;
#8702=LINE ( 'NONE', #12214, #15748 ) ;
#8710=DIRECTION ( 'NONE',  ( 0.7071067811865532349, -0.7071067811865416886, -1.565905175853764455E-16 ) ) ;
#8718=CIRCLE ( 'NONE', #16962, 4.500000000000031974 ) ;
#8720=ORIENTED_EDGE ( 'NONE', *, *, #16417, .T. ) ;
#8729=CARTESIAN_POINT ( 'NONE',  ( -50.65685424949267457, -7.200000000000071232, -8.000000000000007105 ) ) ;
#8737=FACE_OUTER_BOUND ( 'NONE', #19519, .T. ) ;
#8738=AXIS2_PLACEMENT_3D ( 'NONE', #16041, #12516, #7014 ) ;
#8755=ORIENTED_EDGE ( 'NONE', *, *, #7084, .F. ) ;
#8756=VECTOR ( 'NONE', #3925, 1000.000000000000000 ) ;
#8758=AXIS2_PLACEMENT_3D ( 'NONE', #2354, #6013, #5892 ) ;
#8761=DIRECTION ( 'NONE',  ( 0.7071067811865457964, -0.7071067811865492381, 0.000000000000000000 ) ) ;
#8762=VERTEX_POINT ( 'NONE', #1672 ) ;
#8772=DIRECTION ( 'NONE',  ( 2.013525853228507892E-32, 6.902532920683810383E-31, -1.000000000000000000 ) ) ;
#8776=VECTOR ( 'NONE', #10346, 1000.000000000000000 ) ;
#8778=CIRCLE ( 'NONE', #11379, 0.5000000000000049960 ) ;
#8779=ORIENTED_EDGE ( 'NONE', *, *, #21882, .F. ) ;
#8785=ORIENTED_EDGE ( 'NONE', *, *, #18878, .F. ) ;
#8786=ORIENTED_EDGE ( 'NONE', *, *, #18570, .T. ) ;
#8793=AXIS2_PLACEMENT_3D ( 'NONE', #6517, #10042, #1225 ) ;
#8796=FACE_OUTER_BOUND ( 'NONE', #19702, .T. ) ;
#8817=CARTESIAN_POINT ( 'NONE',  ( -50.65685424949270299, 7.200000000000025935, 7.500000000000062172 ) ) ;
#8829=ADVANCED_FACE ( 'NONE', ( #12362 ), #14366, .F. ) ;
#8834=EDGE_CURVE ( 'NONE', #5817, #9446, #23212, .T. ) ;
#8838=EDGE_CURVE ( 'NONE', #4291, #4366, #4239, .T. ) ;
#8842=AXIS2_PLACEMENT_3D ( 'NONE', #15383, #11969, #9990 ) ;
#8848=ORIENTED_EDGE ( 'NONE', *, *, #17990, .T. ) ;
#8849=ORIENTED_EDGE ( 'NONE', *, *, #21171, .T. ) ;
#8852=DIRECTION ( 'NONE',  ( 1.550910762415566494E-16, 1.000000000000000000, -8.135128085091684243E-31 ) ) ;
#8858=CARTESIAN_POINT ( 'NONE',  ( -6.000000000000088818, 1.999999999999960032, -17.72029585817558228 ) ) ;
#8859=DIRECTION ( 'NONE',  ( -2.013525853228507892E-32, -6.902532920683810383E-31, 1.000000000000000000 ) ) ;
#8864=AXIS2_PLACEMENT_3D ( 'NONE', #4226, #20602, #2474 ) ;
#8867=CARTESIAN_POINT ( 'NONE',  ( -65.55642023346347003, 2.700000000000056577, -11.87813525200320797 ) ) ;
#8869=ORIENTED_EDGE ( 'NONE', *, *, #6942, .T. ) ;
#8871=ORIENTED_EDGE ( 'NONE', *, *, #21894, .F. ) ;
#8872=ORIENTED_EDGE ( 'NONE', *, *, #21755, .F. ) ;
#8874=ORIENTED_EDGE ( 'NONE', *, *, #764, .F. ) ;
#8875=ORIENTED_EDGE ( 'NONE', *, *, #16953, .F. ) ;
#8878=CIRCLE ( 'NONE', #2861, 5.500000000000046185 ) ;
#8889=EDGE_CURVE ( 'NONE', #15940, #16720, #5761, .T. ) ;
#8895=AXIS2_PLACEMENT_3D ( 'NONE', #7697, #2394, #20286 ) ;
#8900=ORIENTED_EDGE ( 'NONE', *, *, #7419, .T. ) ;
#8905=AXIS2_PLACEMENT_3D ( 'NONE', #12379, #10505, #14382 ) ;
#8913=CARTESIAN_POINT ( 'NONE',  ( -47.82842712474646873, -4.371572875253880497, -7.500000000000034639 ) ) ;
#8918=CARTESIAN_POINT ( 'NONE',  ( -66.55000000000046612, -7.593235069856354823E-14, -2.000000000000001776 ) ) ;
#8929=VERTEX_POINT ( 'NONE', #13184 ) ;
#8934=EDGE_CURVE ( 'NONE', #10146, #16720, #14785, .T. ) ;
#8936=DIRECTION ( 'NONE',  ( 2.220446049250313081E-16, -1.000000000000000000, 7.025792437124636392E-31 ) ) ;
#8937=ADVANCED_FACE ( 'NONE', ( #22006 ), #5787, .T. ) ;
#8941=EDGE_LOOP ( 'NONE', ( #8848, #11487 ) ) ;
#8953=ADVANCED_FACE ( 'NONE', ( #9649 ), #11063, .T. ) ;
#8960=AXIS2_PLACEMENT_3D ( 'NONE', #11771, #19298, #20726 ) ;
#8968=( GEOMETRIC_REPRESENTATION_CONTEXT ( 3 ) GLOBAL_UNCERTAINTY_ASSIGNED_CONTEXT ( ( #7908 ) ) GLOBAL_UNIT_ASSIGNED_CONTEXT ( ( #7850, #18663, #2548 ) ) REPRESENTATION_CONTEXT ( 'NONE', 'WORKASPACE' ) );
#8971=VECTOR ( 'NONE', #16927, 1000.000000000000227 ) ;
#8987=ORIENTED_EDGE ( 'NONE', *, *, #4369, .T. ) ;
#8989=ORIENTED_EDGE ( 'NONE', *, *, #12969, .T. ) ;
#8997=ORIENTED_EDGE ( 'NONE', *, *, #16109, .F. ) ;
#9008=DIRECTION ( 'NONE',  ( -2.220446049250313081E-16, 1.000000000000000000, -7.025792437124636392E-31 ) ) ;
#9010=CARTESIAN_POINT ( 'NONE',  ( -65.47859922179024750, -3.200000000000088107, -11.38422848940301435 ) ) ;
#9014=DIRECTION ( 'NONE',  ( 1.000000000000000000, 2.220446049250313081E-16, 3.469446951953592101E-15 ) ) ;
#9017=ORIENTED_EDGE ( 'NONE', *, *, #22824, .T. ) ;
#9029=FACE_OUTER_BOUND ( 'NONE', #13670, .T. ) ;
#9030=AXIS2_PLACEMENT_3D ( 'NONE', #16734, #12871, #12991 ) ;
#9035=DIRECTION ( 'NONE',  ( -0.7071067811865485719, 0.7071067811865464625, 1.010793663541191485E-16 ) ) ;
#9038=DIRECTION ( 'NONE',  ( 1.000000000000000000, 0.000000000000000000, 0.000000000000000000 ) ) ;
#9042=ORIENTED_EDGE ( 'NONE', *, *, #14392, .F. ) ;
#9044=ORIENTED_EDGE ( 'NONE', *, *, #14260, .F. ) ;
#9053=EDGE_CURVE ( 'NONE', #6614, #19105, #17043, .T. ) ;
#9063=EDGE_LOOP ( 'NONE', ( #5846, #6158, #5460, #9330 ) ) ;
#9066=ORIENTED_EDGE ( 'NONE', *, *, #19882, .T. ) ;
#9079=DIRECTION ( 'NONE',  ( 1.550910762415566494E-16, 1.000000000000000000, -8.135128085091684243E-31 ) ) ;
#9081=LINE ( 'NONE', #9202, #15892 ) ;
#9085=DIRECTION ( 'NONE',  ( -2.013525853228518840E-32, 6.779273404243028164E-31, -1.000000000000000000 ) ) ;
#9092=CARTESIAN_POINT ( 'NONE',  ( -43.46238456605041023, -4.919238815542528620, -7.500000000000007105 ) ) ;
#9098=VERTEX_POINT ( 'NONE', #6706 ) ;
#9100=VERTEX_POINT ( 'NONE', #15516 ) ;
#9111=CARTESIAN_POINT ( 'NONE',  ( -6.000000000000088818, -8.000000000000042633, 8.000000000000062172 ) ) ;
#9112=AXIS2_PLACEMENT_3D ( 'NONE', #17107, #9836, #15352 ) ;
#9114=DIRECTION ( 'NONE',  ( 0.1556420233463076119, 0.000000000000000000, 0.9878135252003121813 ) ) ;
#9116=LINE ( 'NONE', #15929, #11010 ) ;
#9117=ADVANCED_FACE ( 'NONE', ( #13533 ), #6592, .F. ) ;
#9118=LINE ( 'NONE', #7141, #15507 ) ;
#9122=DIRECTION ( 'NONE',  ( 1.000000000000000000, -1.389842848855773367E-62, 2.013525853228507618E-32 ) ) ;
#9123=DIRECTION ( 'NONE',  ( 2.013525853228507892E-32, 6.902532920683810383E-31, -1.000000000000000000 ) ) ;
#9128=TOROIDAL_SURFACE ( 'NONE', #8738, 5.500000000000007994, 0.5000000000000000000 ) ;
#9130=ORIENTED_EDGE ( 'NONE', *, *, #18929, .F. ) ;
#9131=CIRCLE ( 'NONE', #1241, 0.8000000000000090372 ) ;
#9134=VERTEX_POINT ( 'NONE', #21061 ) ;
#9137=EDGE_LOOP ( 'NONE', ( #8785, #8786, #2646, #19928 ) ) ;
#9142=DIRECTION ( 'NONE',  ( -2.013525853228507892E-32, -6.902532920683810383E-31, 1.000000000000000000 ) ) ;
#9153=CARTESIAN_POINT ( 'NONE',  ( -42.54314575050793934, -4.000000000000021316, 7.500000000000062172 ) ) ;
#9161=AXIS2_PLACEMENT_3D ( 'NONE', #5483, #20371, #9122 ) ;
#9163=ORIENTED_EDGE ( 'NONE', *, *, #18652, .T. ) ;
#9168=ORIENTED_EDGE ( 'NONE', *, *, #10839, .F. ) ;
#9169=PLANE ( 'NONE',  #3162 ) ;
#9172=VERTEX_POINT ( 'NONE', #3183 ) ;
#9189=CIRCLE ( 'NONE', #22348, 5.500000000000033751 ) ;
#9190=ORIENTED_EDGE ( 'NONE', *, *, #16456, .F. ) ;
#9191=ORIENTED_EDGE ( 'NONE', *, *, #3528, .T. ) ;
#9202=CARTESIAN_POINT ( 'NONE',  ( -95.70000000000069917, 0.5000000000000073275, 8.000000000000090594 ) ) ;
#9206=CARTESIAN_POINT ( 'NONE',  ( -56.54644007500109382, -0.5000000000001045830, -8.666666666666655416 ) ) ;
#9210=DIRECTION ( 'NONE',  ( -2.220446049250313081E-16, 1.000000000000000000, -7.025792437124636392E-31 ) ) ;
#9221=ORIENTED_EDGE ( 'NONE', *, *, #15423, .T. ) ;
#9240=EDGE_CURVE ( 'NONE', #9100, #1329, #5778, .T. ) ;
#9244=ORIENTED_EDGE ( 'NONE', *, *, #16023, .F. ) ;
#9246=VECTOR ( 'NONE', #22742, 1000.000000000000000 ) ;
#9247=ORIENTED_EDGE ( 'NONE', *, *, #14867, .T. ) ;
#9254=DIRECTION ( 'NONE',  ( -2.013525853228507892E-32, -6.902532920683810383E-31, 1.000000000000000000 ) ) ;
#9258=AXIS2_PLACEMENT_3D ( 'NONE', #21738, #12663, #10676 ) ;
#9259=DIRECTION ( 'NONE',  ( 0.5833333333333320381, 1.429810390713075314E-30, -0.8122328620674146293 ) ) ;
#9260=DIRECTION ( 'NONE',  ( 0.000000000000000000, 0.000000000000000000, -1.000000000000000000 ) ) ;
#9261=DIRECTION ( 'NONE',  ( 1.550910762415566494E-16, 1.000000000000000000, -8.135128085091684243E-31 ) ) ;
#9264=DIRECTION ( 'NONE',  ( 2.013525853228507892E-32, 6.902532920683810383E-31, -1.000000000000000000 ) ) ;
#9267=DIRECTION ( 'NONE',  ( 1.000000000000000000, -1.550910762415513985E-16, -3.012982189080959477E-32 ) ) ;
#9270=CARTESIAN_POINT ( 'NONE',  ( -43.10883117545713361, 4.565685424949256443, 8.000000000000035527 ) ) ;
#9275=CARTESIAN_POINT ( 'NONE',  ( -6.000000000000088818, -2.000000000000043521, 7.500000000000076383 ) ) ;
#9283=FACE_OUTER_BOUND ( 'NONE', #16970, .T. ) ;
#9299=VERTEX_POINT ( 'NONE', #4092 ) ;
#9306=DIRECTION ( 'NONE',  ( -2.013525853228507892E-32, -6.902532920683810383E-31, 1.000000000000000000 ) ) ;
#9311=CIRCLE ( 'NONE', #4048, 4.000000000000023981 ) ;
#9317=DIRECTION ( 'NONE',  ( 1.107262168541282614E-16, -1.107262168541365321E-16, 1.000000000000000000 ) ) ;
#9323=FACE_OUTER_BOUND ( 'NONE', #14073, .T. ) ;
#9327=AXIS2_PLACEMENT_3D ( 'NONE', #17231, #9837, #18778 ) ;
#9330=ORIENTED_EDGE ( 'NONE', *, *, #7092, .F. ) ;
#9343=VECTOR ( 'NONE', #220, 1000.000000000000000 ) ;
#9352=DIRECTION ( 'NONE',  ( 0.2405376366294550983, 0.000000000000000000, -0.9706398123736303951 ) ) ;
#9368=VERTEX_POINT ( 'NONE', #7516 ) ;
#9377=DIRECTION ( 'NONE',  ( 0.7071067811865535679, -0.7071067811865414665, 0.000000000000000000 ) ) ;
#9380=ADVANCED_FACE ( 'NONE', ( #7862 ), #9169, .T. ) ;
#9396=ORIENTED_EDGE ( 'NONE', *, *, #3592, .T. ) ;
#9397=VECTOR ( 'NONE', #10978, 1000.000000000000000 ) ;
#9400=ADVANCED_FACE ( 'NONE', ( #2446 ), #22098, .T. ) ;
#9422=ORIENTED_EDGE ( 'NONE', *, *, #10091, .T. ) ;
#9428=VECTOR ( 'NONE', #13538, 1000.000000000000000 ) ;
#9429=CARTESIAN_POINT ( 'NONE',  ( -6.000000000000074607, 1.999999999999960032, 7.500000000000062172 ) ) ;
#9440=CARTESIAN_POINT ( 'NONE',  ( -6.000000000000074607, 4.799999999999964295, 7.500000000000062172 ) ) ;
#9444=CIRCLE ( 'NONE', #15444, 3.500000000000023981 ) ;
#9446=VERTEX_POINT ( 'NONE', #2562 ) ;
#9450=ORIENTED_EDGE ( 'NONE', *, *, #22711, .T. ) ;
#9452=VERTEX_POINT ( 'NONE', #8214 ) ;
#9457=DIRECTION ( 'NONE',  ( -1.000000000000000000, 0.000000000000000000, 0.000000000000000000 ) ) ;
#9460=DIRECTION ( 'NONE',  ( -2.013525853228507892E-32, -6.902532920683810383E-31, 1.000000000000000000 ) ) ;
#9466=CARTESIAN_POINT ( 'NONE',  ( -95.20000000000065654, -3.200000000000064126, -2.000000000000001776 ) ) ;
#9473=ORIENTED_EDGE ( 'NONE', *, *, #1645, .F. ) ;
#9486=CARTESIAN_POINT ( 'NONE',  ( -6.866595637048056311, 1.110223024625156540E-13, 27.70872448147268585 ) ) ;
#9495=PLANE ( 'NONE',  #14593 ) ;
#9501=CARTESIAN_POINT ( 'NONE',  ( -52.60445557845683595, -2.775557561562891351E-14, 15.85914177512520773 ) ) ;
#9504=AXIS2_PLACEMENT_3D ( 'NONE', #19296, #18010, #15989 ) ;
#9505=ORIENTED_EDGE ( 'NONE', *, *, #1757, .F. ) ;
#9506=CIRCLE ( 'NONE', #21550, 0.5000000000000029976 ) ;
#9510=CYLINDRICAL_SURFACE ( 'NONE', #21518, 0.5000000000000000000 ) ;
#9515=DIRECTION ( 'NONE',  ( -1.000000000000000000, -1.700709290173333260E-16, 0.000000000000000000 ) ) ;
#9518=DIRECTION ( 'NONE',  ( 1.424116703980846297E-16, -1.000000000000000000, 6.656013887802287108E-31 ) ) ;
#9529=TOROIDAL_SURFACE ( 'NONE', #17387, 1.300000000000000711, 0.5000000000000000000 ) ;
#9533=ADVANCED_FACE ( 'NONE', ( #22564 ), #13624, .T. ) ;
#9537=ORIENTED_EDGE ( 'NONE', *, *, #943, .F. ) ;
#9546=DIRECTION ( 'NONE',  ( -1.000000000000000000, 0.000000000000000000, 0.000000000000000000 ) ) ;
#9547=DIRECTION ( 'NONE',  ( 0.7071067811865457964, 0.7071067811865492381, 0.000000000000000000 ) ) ;
#9549=ADVANCED_FACE ( 'NONE', ( #8451 ), #17250, .T. ) ;
#9559=CARTESIAN_POINT ( 'NONE',  ( -50.65685424949271720, -0.5000000000001045830, 7.500000000000076383 ) ) ;
#9575=VERTEX_POINT ( 'NONE', #4898 ) ;
#9585=DIRECTION ( 'NONE',  ( 0.000000000000000000, 0.000000000000000000, 1.000000000000000000 ) ) ;
#9586=SURFACE_STYLE_FILL_AREA ( #20293 ) ;
#9589=ORIENTED_EDGE ( 'NONE', *, *, #883, .T. ) ;
#9596=ORIENTED_EDGE ( 'NONE', *, *, #21040, .T. ) ;
#9598=EDGE_CURVE ( 'NONE', #1919, #4144, #2716, .T. ) ;
#9601=LINE ( 'NONE', #1014, #1620 ) ;
#9612=LINE ( 'NONE', #11256, #12523 ) ;
#9615=( NAMED_UNIT ( * ) PLANE_ANGLE_UNIT ( ) SI_UNIT ( $, .RADIAN. ) );
#9616=DIRECTION ( 'NONE',  ( 0.7071067811865460184, -0.7071067811865490160, -1.010793663541200360E-16 ) ) ;
#9629=DIRECTION ( 'NONE',  ( 0.1556420233463033653, 0.000000000000000000, 0.9878135252003128475 ) ) ;
#9633=DIRECTION ( 'NONE',  ( -0.9878135252003118483, -1.429810390713075314E-30, 0.1556420233463089442 ) ) ;
#9634=CARTESIAN_POINT ( 'NONE',  ( -6.000000000000116351, 5.299999999999957190, -7.500000000000062172 ) ) ;
#9635=FACE_OUTER_BOUND ( 'NONE', #6754, .T. ) ;
#9649=FACE_OUTER_BOUND ( 'NONE', #2055, .T. ) ;
#9667=DIRECTION ( 'NONE',  ( -1.000000000000000000, 9.957992501029406452E-17, 2.655250634480538332E-32 ) ) ;
#9669=VERTEX_POINT ( 'NONE', #19609 ) ;
#9671=EDGE_CURVE ( 'NONE', #21212, #6874, #6109, .T. ) ;
#9672=EDGE_CURVE ( 'NONE', #19569, #16720, #3273, .T. ) ;
#9673=ORIENTED_EDGE ( 'NONE', *, *, #3757, .T. ) ;
#9687=CARTESIAN_POINT ( 'NONE',  ( -50.65685424949267457, -2.700000000000091216, -7.500000000000034639 ) ) ;
#9688=CARTESIAN_POINT ( 'NONE',  ( -2.700000000000063238, 4.799999999999935874, 8.000000000000062172 ) ) ;
#9691=ADVANCED_FACE ( 'NONE', ( #15950 ), #16224, .T. ) ;
#9693=VECTOR ( 'NONE', #8772, 1000.000000000000000 ) ;
#9697=DIRECTION ( 'NONE',  ( -0.9706398123736330597, -2.155253336630096709E-16, -0.2405376366294442736 ) ) ;
#9715=AXIS2_PLACEMENT_3D ( 'NONE', #18116, #1539, #12705 ) ;
#9733=LINE ( 'NONE', #8076, #21298 ) ;
#9739=EDGE_CURVE ( 'NONE', #12565, #22996, #316, .T. ) ;
#9742=EDGE_LOOP ( 'NONE', ( #12865, #12823, #15685, #2616 ) ) ;
#9749=AXIS2_PLACEMENT_3D ( 'NONE', #7273, #16309, #6798 ) ;
#9755=DIRECTION ( 'NONE',  ( -1.550910762415566494E-16, -1.000000000000000000, 8.135128085091684243E-31 ) ) ;
#9758=DIRECTION ( 'NONE',  ( -1.000000000000000000, 2.833381677428764831E-14, 0.000000000000000000 ) ) ;
#9772=CARTESIAN_POINT ( 'NONE',  ( -49.51923881554284890, -1.137615433949877630, 8.000000000000076383 ) ) ;
#9788=VERTEX_POINT ( 'NONE', #5731 ) ;
#9791=ADVANCED_FACE ( 'NONE', ( #554 ), #18204, .T. ) ;
#9792=ORIENTED_EDGE ( 'NONE', *, *, #21051, .T. ) ;
#9793=EDGE_LOOP ( 'NONE', ( #18593, #307, #309, #12594 ) ) ;
#9794=AXIS2_PLACEMENT_3D ( 'NONE', #18952, #22482, #17166 ) ;
#9804=DIRECTION ( 'NONE',  ( 2.013525853228507892E-32, 6.902532920683810383E-31, -1.000000000000000000 ) ) ;
#9813=LINE ( 'NONE', #18867, #9343 ) ;
#9816=CARTESIAN_POINT ( 'NONE',  ( -65.47859922179033276, 2.700000000000056577, -11.38422848940298593 ) ) ;
#9822=ORIENTED_EDGE ( 'NONE', *, *, #22898, .T. ) ;
#9825=ORIENTED_EDGE ( 'NONE', *, *, #5661, .T. ) ;
#9833=DIRECTION ( 'NONE',  ( 0.000000000000000000, 1.000000000000000000, 0.000000000000000000 ) ) ;
#9836=DIRECTION ( 'NONE',  ( 1.424116703980846297E-16, -1.000000000000000000, 6.656013887802287108E-31 ) ) ;
#9837=DIRECTION ( 'NONE',  ( -2.013525853228507892E-32, -6.902532920683810383E-31, 1.000000000000000000 ) ) ;
#9843=ORIENTED_EDGE ( 'NONE', *, *, #14869, .F. ) ;
#9855=CARTESIAN_POINT ( 'NONE',  ( -50.65685424949274562, -1.040834085586084257E-13, 8.000000000000062172 ) ) ;
#9869=EDGE_CURVE ( 'NONE', #2652, #22532, #9601, .T. ) ;
#9871=AXIS2_PLACEMENT_3D ( 'NONE', #9855, #1041, #22560 ) ;
#9874=DIRECTION ( 'NONE',  ( 1.550910762415566494E-16, 1.000000000000000000, -8.135128085091684243E-31 ) ) ;
#9875=CARTESIAN_POINT ( 'NONE',  ( -55.25320565519142946, -4.163336342344337027E-14, 8.000000000000076383 ) ) ;
#9882=EDGE_LOOP ( 'NONE', ( #511, #11333, #11288, #17072 ) ) ;
#9884=AXIS2_PLACEMENT_3D ( 'NONE', #18653, #13718, #20669 ) ;
#9887=ORIENTED_EDGE ( 'NONE', *, *, #5663, .F. ) ;
#9888=CARTESIAN_POINT ( 'NONE',  ( -6.000000000000047073, -4.800000000000006040, 8.000000000000090594 ) ) ;
#9889=CARTESIAN_POINT ( 'NONE',  ( -55.25320565519148630, -0.5000000000000281997, 7.500000000000007105 ) ) ;
#9894=CARTESIAN_POINT ( 'NONE',  ( -64.00000000000045475, -7.632783294297951215E-14, -2.000000000000001776 ) ) ;
#9900=VECTOR ( 'NONE', #21189, 1000.000000000000114 ) ;
#9901=CYLINDRICAL_SURFACE ( 'NONE', #2727, 0.5000000000000037748 ) ;
#9904=AXIS2_PLACEMENT_3D ( 'NONE', #20250, #7657, #11521 ) ;
#9914=ORIENTED_EDGE ( 'NONE', *, *, #16692, .F. ) ;
#9917=VERTEX_POINT ( 'NONE', #4290 ) ;
#9926=LINE ( 'NONE', #4266, #18782 ) ;
#9933=DIRECTION ( 'NONE',  ( -2.220446049250313081E-16, 1.000000000000000000, -7.025792437124636392E-31 ) ) ;
#9938=FACE_OUTER_BOUND ( 'NONE', #18196, .T. ) ;
#9939=CIRCLE ( 'NONE', #5431, 7.200000000000046363 ) ;
#9949=ORIENTED_EDGE ( 'NONE', *, *, #16944, .F. ) ;
#9950=EDGE_CURVE ( 'NONE', #19389, #4887, #3120, .T. ) ;
#9953=AXIS2_PLACEMENT_3D ( 'NONE', #12584, #19769, #3649 ) ;
#9955=ORIENTED_EDGE ( 'NONE', *, *, #761, .F. ) ;
#9968=ORIENTED_EDGE ( 'NONE', *, *, #484, .F. ) ;
#9969=EDGE_CURVE ( 'NONE', #16222, #18640, #4528, .T. ) ;
#9984=DIRECTION ( 'NONE',  ( -0.7071067811865457964, 0.7071067811865492381, 0.000000000000000000 ) ) ;
#9986=DIRECTION ( 'NONE',  ( -1.000000000000000000, 1.550910762415566494E-16, 6.133276141584333908E-48 ) ) ;
#9990=DIRECTION ( 'NONE',  ( 0.2405376366294273427, 0.000000000000000000, -0.9706398123736372785 ) ) ;
#9991=EDGE_CURVE ( 'NONE', #16222, #22909, #5756, .T. ) ;
#9999=ADVANCED_FACE ( 'NONE', ( #19349 ), #3245, .T. ) ;
#10007=CARTESIAN_POINT ( 'NONE',  ( -64.00000000000045475, -7.632783294297951215E-14, -2.000000000000001776 ) ) ;
#10013=DIRECTION ( 'NONE',  ( -1.000000000000000000, 0.000000000000000000, 0.000000000000000000 ) ) ;
#10027=ORIENTED_EDGE ( 'NONE', *, *, #22163, .T. ) ;
#10029=EDGE_LOOP ( 'NONE', ( #9422, #18703, #7835, #20048 ) ) ;
#10030=ORIENTED_EDGE ( 'NONE', *, *, #15869, .F. ) ;
#10036=CARTESIAN_POINT ( 'NONE',  ( -6.000000000000130562, 7.499999999999958256, -8.000000000000035527 ) ) ;
#10040=CARTESIAN_POINT ( 'NONE',  ( -95.20000000000064233, 2.700000000000014833, 1.000000000000014655 ) ) ;
#10042=DIRECTION ( 'NONE',  ( -0.9878135252003120703, -1.079983486989479408E-15, 0.1556420233463082226 ) ) ;
#10046=CARTESIAN_POINT ( 'NONE',  ( -50.65685424949277404, -1.040834085586084257E-13, -7.500000000000062172 ) ) ;
#10051=CIRCLE ( 'NONE', #7418, 7.200000000000046363 ) ;
#10059=CARTESIAN_POINT ( 'NONE',  ( -95.20000000000052864, -3.200000000000064126, 1.000000000000000888 ) ) ;
#10062=ORIENTED_EDGE ( 'NONE', *, *, #19894, .T. ) ;
#10064=CARTESIAN_POINT ( 'NONE',  ( -42.54314575050799618, 3.999999999999996447, 8.000000000000035527 ) ) ;
#10070=CARTESIAN_POINT ( 'NONE',  ( -65.00000000000052580, 5.551115123125782702E-14, 3.000000000000002665 ) ) ;
#10072=CIRCLE ( 'NONE', #7823, 2.800000000000017142 ) ;
#10073=DIRECTION ( 'NONE',  ( -2.013525853228507892E-32, -6.902532920683810383E-31, 1.000000000000000000 ) ) ;
#10074=CARTESIAN_POINT ( 'NONE',  ( -50.65685424949277404, 3.200000000000022382, 8.000000000000021316 ) ) ;
#10075=EDGE_CURVE ( 'NONE', #20271, #15092, #9131, .T. ) ;
#10077=VECTOR ( 'NONE', #19614, 1000.000000000000000 ) ;
#10083=AXIS2_PLACEMENT_3D ( 'NONE', #1088, #4717, #11886 ) ;
#10087=ORIENTED_EDGE ( 'NONE', *, *, #20199, .F. ) ;
#10091=EDGE_CURVE ( 'NONE', #5077, #477, #11378, .T. ) ;
#10093=ORIENTED_EDGE ( 'NONE', *, *, #78, .T. ) ;
#10107=CARTESIAN_POINT ( 'NONE',  ( -55.05572809000122447, -3.200000000000088107, -10.00000000000006395 ) ) ;
#10110=FACE_OUTER_BOUND ( 'NONE', #5375, .T. ) ;
#10119=EDGE_CURVE ( 'NONE', #19838, #5921, #23042, .T. ) ;
#10121=ORIENTED_EDGE ( 'NONE', *, *, #11836, .T. ) ;
#10125=VERTEX_POINT ( 'NONE', #3125 ) ;
#10126=CARTESIAN_POINT ( 'NONE',  ( -50.65685424949278826, 1.387778780781445676E-14, -7.500000000000034639 ) ) ;
#10129=DIRECTION ( 'NONE',  ( 0.000000000000000000, -6.938893903907186568E-15, 1.000000000000000000 ) ) ;
#10133=DIRECTION ( 'NONE',  ( 0.7071067811865457964, -0.7071067811865492381, 0.000000000000000000 ) ) ;
#10135=DIRECTION ( 'NONE',  ( -1.000000000000000000, 1.550910762415526064E-16, 0.000000000000000000 ) ) ;
#10141=VERTEX_POINT ( 'NONE', #18061 ) ;
#10146=VERTEX_POINT ( 'NONE', #21940 ) ;
#10147=DIRECTION ( 'NONE',  ( -1.000000000000000000, 1.424116703980815236E-16, 2.931272055834072749E-32 ) ) ;
#10149=CIRCLE ( 'NONE', #15764, 5.500000000000046185 ) ;
#10154=DIRECTION ( 'NONE',  ( -2.220446049250313081E-16, 1.000000000000000000, -7.025792437124636392E-31 ) ) ;
#10158=EDGE_CURVE ( 'NONE', #20601, #14402, #4986, .T. ) ;
#10159=CARTESIAN_POINT ( 'NONE',  ( -55.05572809000125289, 2.700000000000021938, -10.00000000000006395 ) ) ;
#10167=ORIENTED_EDGE ( 'NONE', *, *, #7084, .T. ) ;
#10169=ORIENTED_EDGE ( 'NONE', *, *, #6951, .T. ) ;
#10171=FACE_OUTER_BOUND ( 'NONE', #3797, .T. ) ;
#10172=DIRECTION ( 'NONE',  ( 1.281898970984144184E-30, 1.000000000000000000, 6.938893903907263876E-15 ) ) ;
#10186=CARTESIAN_POINT ( 'NONE',  ( -50.65685424949274562, 2.700000000000021938, -8.000000000000062172 ) ) ;
#10190=AXIS2_PLACEMENT_3D ( 'NONE', #18928, #11386, #21159 ) ;
#10192=EDGE_LOOP ( 'NONE', ( #21443, #4361, #8874, #3534 ) ) ;
#10199=CARTESIAN_POINT ( 'NONE',  ( -67.28510754798014659, -3.200000000000105427, 12.22107821754958579 ) ) ;
#10200=CARTESIAN_POINT ( 'NONE',  ( -42.54314575050793934, 7.999999999999992895, 7.500000000000062172 ) ) ;
#10211=EDGE_CURVE ( 'NONE', #11574, #8147, #12514, .T. ) ;
#10214=EDGE_CURVE ( 'NONE', #7485, #21952, #21907, .T. ) ;
#10223=EDGE_CURVE ( 'NONE', #20271, #8929, #14420, .T. ) ;
#10237=CARTESIAN_POINT ( 'NONE',  ( -89.70000000000057128, -0.5000000000000628386, -2.000000000000001776 ) ) ;
#10245=ORIENTED_EDGE ( 'NONE', *, *, #18447, .T. ) ;
#10252=ADVANCED_FACE ( 'NONE', ( #6712 ), #9529, .T. ) ;
#10256=EDGE_CURVE ( 'NONE', #9446, #4139, #17406, .T. ) ;
#10260=TOROIDAL_SURFACE ( 'NONE', #4611, 5.500000000000003553, 0.5000000000000000000 ) ;
#10262=AXIS2_PLACEMENT_3D ( 'NONE', #12099, #11990, #6596 ) ;
#10263=DIRECTION ( 'NONE',  ( -2.220446049250313081E-16, 1.000000000000000000, -7.025792437124636392E-31 ) ) ;
#10265=AXIS2_PLACEMENT_3D ( 'NONE', #1551, #10598, #14488 ) ;
#10274=EDGE_LOOP ( 'NONE', ( #6876, #17242, #13817, #3240 ) ) ;
#10275=VECTOR ( 'NONE', #21260, 1000.000000000000114 ) ;
#10277=EDGE_LOOP ( 'NONE', ( #16402, #1352, #3029, #12183 ) ) ;
#10279=AXIS2_PLACEMENT_3D ( 'NONE', #814, #1051, #9986 ) ;
#10282=AXIS2_PLACEMENT_3D ( 'NONE', #14110, #8936, #8 ) ;
#10284=EDGE_LOOP ( 'NONE', ( #6590, #21241, #14468, #6818 ) ) ;
#10291=DIRECTION ( 'NONE',  ( -1.550910762415566494E-16, -1.000000000000000000, 8.135128085091684243E-31 ) ) ;
#10298=VECTOR ( 'NONE', #2278, 1000.000000000000000 ) ;
#10322=FACE_OUTER_BOUND ( 'NONE', #15654, .T. ) ;
#10325=ADVANCED_FACE ( 'NONE', ( #21067 ), #6530, .T. ) ;
#10326=DIRECTION ( 'NONE',  ( -1.550910762415566494E-16, -1.000000000000000000, 8.135128085091684243E-31 ) ) ;
#10327=VECTOR ( 'NONE', #8710, 1000.000000000000114 ) ;
#10328=DIRECTION ( 'NONE',  ( 0.7071067811865490160, 0.7071067811865460184, 1.565905175853766674E-16 ) ) ;
#10332=CARTESIAN_POINT ( 'NONE',  ( -45.91923881554277642, -2.462384566050232593, 8.000000000000047962 ) ) ;
#10335=ORIENTED_EDGE ( 'NONE', *, *, #16432, .F. ) ;
#10339=AXIS2_PLACEMENT_3D ( 'NONE', #21063, #6948, #22951 ) ;
#10344=DIRECTION ( 'NONE',  ( -1.000000000000000000, 1.389842848855773367E-62, -2.013525853228507892E-32 ) ) ;
#10346=DIRECTION ( 'NONE',  ( -1.331202777560457422E-30, -1.000000000000000000, 7.395570986446985676E-31 ) ) ;
#10350=ADVANCED_FACE ( 'NONE', ( #22273 ), #13104, .F. ) ;
#10354=CARTESIAN_POINT ( 'NONE',  ( -45.01801948466091829, 6.474873734152911453, -7.500000000000062172 ) ) ;
#10357=FACE_BOUND ( 'NONE', #20123, .T. ) ;
#10358=EDGE_CURVE ( 'NONE', #5921, #7127, #1307, .T. ) ;
#10363=ORIENTED_EDGE ( 'NONE', *, *, #3328, .F. ) ;
#10364=CIRCLE ( 'NONE', #8122, 0.5000000000000000000 ) ;
#10370=LINE ( 'NONE', #10720, #19732 ) ;
#10376=FACE_OUTER_BOUND ( 'NONE', #14, .T. ) ;
#10378=ADVANCED_FACE ( 'NONE', ( #13214 ), #11560, .F. ) ;
#10380=FACE_OUTER_BOUND ( 'NONE', #23093, .T. ) ;
#10383=AXIS2_PLACEMENT_3D ( 'NONE', #3599, #19238, #22903 ) ;
#10393=ORIENTED_EDGE ( 'NONE', *, *, #8232, .F. ) ;
#10394=EDGE_LOOP ( 'NONE', ( #786, #12181, #1456, #16539 ) ) ;
#10399=ADVANCED_FACE ( 'NONE', ( #11441 ), #12454, .T. ) ;
#10400=AXIS2_PLACEMENT_3D ( 'NONE', #19102, #17210, #8289 ) ;
#10402=EDGE_CURVE ( 'NONE', #10662, #23066, #18003, .T. ) ;
#10411=CIRCLE ( 'NONE', #665, 0.5000000000000029976 ) ;
#10417=CARTESIAN_POINT ( 'NONE',  ( -43.46238456605044576, 4.919238815542528620, -8.000000000000035527 ) ) ;
#10419=DIRECTION ( 'NONE',  ( 0.2405376366294550983, 0.000000000000000000, -0.9706398123736303951 ) ) ;
#10426=DIRECTION ( 'NONE',  ( -2.013525853228518840E-32, 6.902532920683810383E-31, -1.000000000000000000 ) ) ;
#10427=DIRECTION ( 'NONE',  ( -2.220446049250313081E-16, 1.000000000000000000, -7.025792437124636392E-31 ) ) ;
#10432=VERTEX_POINT ( 'NONE', #12338 ) ;
#10434=CIRCLE ( 'NONE', #3308, 0.5000000000000029976 ) ;
#10443=LINE ( 'NONE', #21626, #10077 ) ;
#10446=ADVANCED_FACE ( 'NONE', ( #19403 ), #12136, .T. ) ;
#10458=ORIENTED_EDGE ( 'NONE', *, *, #461, .T. ) ;
#10472=CARTESIAN_POINT ( 'NONE',  ( -9.714451465470119729E-14, 1.999999999999890754, 8.000000000000090594 ) ) ;
#10474=PLANE ( 'NONE',  #152 ) ;
#10479=CYLINDRICAL_SURFACE ( 'NONE', #9715, 0.5000000000000004441 ) ;
#10481=AXIS2_PLACEMENT_3D ( 'NONE', #11833, #17471, #6772 ) ;
#10485=ORIENTED_EDGE ( 'NONE', *, *, #3509, .T. ) ;
#10488=ORIENTED_EDGE ( 'NONE', *, *, #15535, .F. ) ;
#10500=DIRECTION ( 'NONE',  ( -0.7071067811865457964, 0.7071067811865492381, 0.000000000000000000 ) ) ;
#10505=DIRECTION ( 'NONE',  ( -1.550910762415566494E-16, -1.000000000000000000, 8.135128085091684243E-31 ) ) ;
#10506=FACE_OUTER_BOUND ( 'NONE', #5176, .T. ) ;
#10510=ADVANCED_FACE ( 'NONE', ( #1532 ), #12905, .T. ) ;
#10518=ORIENTED_EDGE ( 'NONE', *, *, #21604, .F. ) ;
#10535=CARTESIAN_POINT ( 'NONE',  ( -55.25320565519140104, -2.700000000000049472, 7.500000000000047962 ) ) ;
#10552=LINE ( 'NONE', #5144, #21292 ) ;
#10562=DIRECTION ( 'NONE',  ( 2.710505431213791653E-16, 1.000000000000000000, -4.807121141190541565E-31 ) ) ;
#10567=ORIENTED_EDGE ( 'NONE', *, *, #20475, .T. ) ;
#10571=ORIENTED_EDGE ( 'NONE', *, *, #22790, .F. ) ;
#10572=EDGE_LOOP ( 'NONE', ( #4362, #4402, #804, #12329 ) ) ;
#10580=CIRCLE ( 'NONE', #7219, 0.5000000000000028866 ) ;
#10581=CIRCLE ( 'NONE', #13595, 0.5000000000000006661 ) ;
#10585=CARTESIAN_POINT ( 'NONE',  ( -90.55603112840523750, -2.700000000000084110, -7.432974388601742533 ) ) ;
#10588=DIRECTION ( 'NONE',  ( 1.000000000000000000, -1.424116703980815236E-16, -2.931272055834072749E-32 ) ) ;
#10589=CARTESIAN_POINT ( 'NONE',  ( -2.700000000000132960, 1.999999999999904521, 8.000000000000076383 ) ) ;
#10590=CARTESIAN_POINT ( 'NONE',  ( -50.65685424949281668, 3.200000000000022382, -7.500000000000089706 ) ) ;
#10593=EDGE_LOOP ( 'NONE', ( #2762, #16405, #22332, #7453 ) ) ;
#10598=DIRECTION ( 'NONE',  ( -2.220446049250313081E-16, 1.000000000000000000, -7.025792437124636392E-31 ) ) ;
#10600=DIRECTION ( 'NONE',  ( -2.013525853228507892E-32, -6.902532920683810383E-31, 1.000000000000000000 ) ) ;
#10603=DIRECTION ( 'NONE',  ( 0.9706398123736329486, -1.505375731439247187E-16, 0.2405376366294442458 ) ) ;
#10605=CARTESIAN_POINT ( 'NONE',  ( -67.40537636629493079, 2.081668171172168513E-14, 12.70639812373644517 ) ) ;
#10615=LINE ( 'NONE', #15786, #7818 ) ;
#10623=ORIENTED_EDGE ( 'NONE', *, *, #18450, .F. ) ;
#10624=ORIENTED_EDGE ( 'NONE', *, *, #17910, .F. ) ;
#10631=AXIS2_PLACEMENT_3D ( 'NONE', #14375, #18142, #5452 ) ;
#10639=EDGE_CURVE ( 'NONE', #21725, #16028, #5409, .T. ) ;
#10646=VECTOR ( 'NONE', #9035, 1000.000000000000114 ) ;
#10648=CYLINDRICAL_SURFACE ( 'NONE', #10665, 4.000000000000014211 ) ;
#10649=AXIS2_PLACEMENT_3D ( 'NONE', #5995, #16444, #14684 ) ;
#10651=TOROIDAL_SURFACE ( 'NONE', #521, 4.500000000000002665, 0.5000000000000000000 ) ;
#10657=CARTESIAN_POINT ( 'NONE',  ( -6.000000000000088818, -2.000000000000043521, -7.500000000000007105 ) ) ;
#10658=DIRECTION ( 'NONE',  ( 0.5833333333333344806, -8.095376221225076634E-15, -0.8122328620674129640 ) ) ;
#10662=VERTEX_POINT ( 'NONE', #21870 ) ;
#10665=AXIS2_PLACEMENT_3D ( 'NONE', #1714, #17705, #7144 ) ;
#10668=CIRCLE ( 'NONE', #3522, 6.000000000000047073 ) ;
#10670=FACE_OUTER_BOUND ( 'NONE', #5951, .T. ) ;
#10673=DIRECTION ( 'NONE',  ( 1.331202777560457422E-30, 1.000000000000000000, -7.395570986446985676E-31 ) ) ;
#10676=DIRECTION ( 'NONE',  ( -1.000000000000000000, 1.550910762415510534E-16, 0.000000000000000000 ) ) ;
#10677=EDGE_CURVE ( 'NONE', #21644, #10770, #22314, .T. ) ;
#10678=DIRECTION ( 'NONE',  ( 1.000000000000000000, 2.168404344970991858E-16, 0.000000000000000000 ) ) ;
#10683=VECTOR ( 'NONE', #2053, 1000.000000000000114 ) ;
#10684=ADVANCED_FACE ( 'NONE', ( #18571 ), #16671, .T. ) ;
#10691=ORIENTED_EDGE ( 'NONE', *, *, #16294, .T. ) ;
#10697=ADVANCED_FACE ( 'NONE', ( #22695 ), #3891, .T. ) ;
#10699=DIRECTION ( 'NONE',  ( 1.550910762415566494E-16, 1.000000000000000000, -8.135128085091684243E-31 ) ) ;
#10702=FACE_OUTER_BOUND ( 'NONE', #9742, .T. ) ;
#10713=VECTOR ( 'NONE', #2948, 1000.000000000000000 ) ;
#10715=ORIENTED_EDGE ( 'NONE', *, *, #8110, .T. ) ;
#10720=CARTESIAN_POINT ( 'NONE',  ( -0.5000000000000837108, 1.999999999999883871, 8.000000000000076383 ) ) ;
#10729=FACE_OUTER_BOUND ( 'NONE', #17454, .T. ) ;
#10736=CIRCLE ( 'NONE', #15980, 0.4999999999999994449 ) ;
#10740=ADVANCED_FACE ( 'NONE', ( #17255 ), #154, .T. ) ;
#10751=PLANE ( 'NONE',  #7311 ) ;
#10755=AXIS2_PLACEMENT_3D ( 'NONE', #9816, #881, #2517 ) ;
#10757=DIRECTION ( 'NONE',  ( 2.013525853228507892E-32, 6.902532920683810383E-31, -1.000000000000000000 ) ) ;
#10769=DIRECTION ( 'NONE',  ( 1.000000000000000000, 2.220446049250313081E-16, -3.656342123407315983E-48 ) ) ;
#10770=VERTEX_POINT ( 'NONE', #20574 ) ;
#10771=ORIENTED_EDGE ( 'NONE', *, *, #22174, .T. ) ;
#10774=ORIENTED_EDGE ( 'NONE', *, *, #20074, .F. ) ;
#10776=ORIENTED_EDGE ( 'NONE', *, *, #7124, .T. ) ;
#10778=EDGE_CURVE ( 'NONE', #8087, #17188, #18190, .T. ) ;
#10791=DIRECTION ( 'NONE',  ( 0.7071067811865534569, 0.7071067811865416886, 1.565905175853764455E-16 ) ) ;
#10796=ORIENTED_EDGE ( 'NONE', *, *, #2964, .F. ) ;
#10799=ORIENTED_EDGE ( 'NONE', *, *, #67, .F. ) ;
#10815=AXIS2_PLACEMENT_3D ( 'NONE', #17556, #3228, #1564 ) ;
#10822=AXIS2_PLACEMENT_3D ( 'NONE', #6867, #1348, #3573 ) ;
#10829=ADVANCED_FACE ( 'NONE', ( #10322 ), #1728, .T. ) ;
#10839=EDGE_CURVE ( 'NONE', #19780, #17901, #19623, .T. ) ;
#10845=AXIS2_PLACEMENT_3D ( 'NONE', #4299, #13144, #20319 ) ;
#10846=FACE_OUTER_BOUND ( 'NONE', #10274, .T. ) ;
#10847=AXIS2_PLACEMENT_3D ( 'NONE', #15559, #9697, #13344 ) ;
#10853=DIRECTION ( 'NONE',  ( -0.7071067811865541231, 0.7071067811865411334, 1.565905175853764948E-16 ) ) ;
#10856=ORIENTED_EDGE ( 'NONE', *, *, #20173, .T. ) ;
#10861=ORIENTED_EDGE ( 'NONE', *, *, #18215, .F. ) ;
#10867=VECTOR ( 'NONE', #3416, 1000.000000000000114 ) ;
#10868=PLANE ( 'NONE',  #20676 ) ;
#10872=FACE_OUTER_BOUND ( 'NONE', #22991, .T. ) ;
#10873=DIRECTION ( 'NONE',  ( -1.000000000000000000, 0.000000000000000000, 0.000000000000000000 ) ) ;
#10877=EDGE_CURVE ( 'NONE', #1743, #9669, #17614, .T. ) ;
#10880=FACE_OUTER_BOUND ( 'NONE', #23089, .T. ) ;
#10881=VECTOR ( 'NONE', #17580, 1000.000000000000227 ) ;
#10882=ORIENTED_EDGE ( 'NONE', *, *, #14353, .T. ) ;
#10883=ORIENTED_EDGE ( 'NONE', *, *, #22036, .F. ) ;
#10886=VERTEX_POINT ( 'NONE', #8676 ) ;
#10888=DIRECTION ( 'NONE',  ( -2.013525853228507892E-32, -6.902532920683810383E-31, 1.000000000000000000 ) ) ;
#10889=DIRECTION ( 'NONE',  ( 4.336808689942045346E-15, -1.000000000000000000, -7.518830502887770522E-31 ) ) ;
#10894=DIRECTION ( 'NONE',  ( 1.000000000000000000, 1.479114197289388027E-30, -2.013525853228518840E-32 ) ) ;
#10895=CARTESIAN_POINT ( 'NONE',  ( -56.87767137932630845, 2.700000000000098321, 8.833333333333415638 ) ) ;
#10896=CARTESIAN_POINT ( 'NONE',  ( -6.000000000000047073, -5.300000000000006040, 8.000000000000090594 ) ) ;
#10904=CARTESIAN_POINT ( 'NONE',  ( -50.65685424949275983, 7.200000000000018829, -8.000000000000007105 ) ) ;
#10921=CIRCLE ( 'NONE', #12814, 10.00000000000006395 ) ;
#10922=CARTESIAN_POINT ( 'NONE',  ( -6.000000000000019540, -4.800000000000006040, 7.500000000000062172 ) ) ;
#10927=ORIENTED_EDGE ( 'NONE', *, *, #13816, .T. ) ;
#10935=EDGE_LOOP ( 'NONE', ( #7225, #14046, #5916, #14136 ) ) ;
#10936=ORIENTED_EDGE ( 'NONE', *, *, #20005, .T. ) ;
#10938=AXIS2_PLACEMENT_3D ( 'NONE', #15295, #4349, #22486 ) ;
#10943=DIRECTION ( 'NONE',  ( 1.000000000000000000, 2.168404344970992105E-16, 0.000000000000000000 ) ) ;
#10944=LINE ( 'NONE', #17666, #7628 ) ;
#10945=DIRECTION ( 'NONE',  ( -1.000000000000000000, -1.479114197289388027E-30, 2.013525853228518840E-32 ) ) ;
#10947=EDGE_CURVE ( 'NONE', #15196, #6879, #3469, .T. ) ;
#10949=DIRECTION ( 'NONE',  ( 2.013525853228507892E-32, 6.902532920683810383E-31, -1.000000000000000000 ) ) ;
#10958=DIRECTION ( 'NONE',  ( -1.000000000000000000, 1.626303258728244079E-16, 0.000000000000000000 ) ) ;
#10959=ORIENTED_EDGE ( 'NONE', *, *, #2522, .T. ) ;
#10966=VERTEX_POINT ( 'NONE', #3499 ) ;
#10976=DIRECTION ( 'NONE',  ( -1.000000000000000000, 0.000000000000000000, 0.000000000000000000 ) ) ;
#10978=DIRECTION ( 'NONE',  ( -1.000000000000000000, -1.424116703980846297E-16, 1.095779650622964657E-32 ) ) ;
#10982=ADVANCED_FACE ( 'NONE', ( #20312 ), #13019, .F. ) ;
#10983=CARTESIAN_POINT ( 'NONE',  ( -90.55603112840523750, -0.5000000000000628386, -7.432974388601742533 ) ) ;
#10991=CARTESIAN_POINT ( 'NONE',  ( -45.37157287525420202, 6.828427124746163202, 7.500000000000089706 ) ) ;
#10995=AXIS2_PLACEMENT_3D ( 'NONE', #11068, #11297, #18478 ) ;
#10997=ORIENTED_EDGE ( 'NONE', *, *, #21959, .F. ) ;
#11001=VERTEX_POINT ( 'NONE', #20084 ) ;
#11009=CARTESIAN_POINT ( 'NONE',  ( -89.70000000000057128, -9.020562075079396891E-14, -2.000000000000001776 ) ) ;
#11010=VECTOR ( 'NONE', #21826, 1000.000000000000000 ) ;
#11011=CYLINDRICAL_SURFACE ( 'NONE', #11981, 0.5000000000000037748 ) ;
#11016=AXIS2_PLACEMENT_3D ( 'NONE', #5087, #8385, #1216 ) ;
#11017=ADVANCED_FACE ( 'NONE', ( #319 ), #12779, .F. ) ;
#11019=DIRECTION ( 'NONE',  ( -1.392757777031969319E-14, -1.000000000000000000, 5.941108692445745160E-30 ) ) ;
#11025=CARTESIAN_POINT ( 'NONE',  ( -45.01801948466080461, -6.474873734152907900, -8.000000000000035527 ) ) ;
#11027=EDGE_CURVE ( 'NONE', #21952, #4281, #18424, .T. ) ;
#11030=AXIS2_PLACEMENT_3D ( 'NONE', #2809, #4442, #17023 ) ;
#11031=VECTOR ( 'NONE', #4170, 1000.000000000000114 ) ;
#11032=CARTESIAN_POINT ( 'NONE',  ( -42.54314575050785407, -7.500000000000020428, 8.000000000000007105 ) ) ;
#11035=DIRECTION ( 'NONE',  ( 1.000000000000000000, 0.000000000000000000, 0.000000000000000000 ) ) ;
#11040=ORIENTED_EDGE ( 'NONE', *, *, #78, .F. ) ;
#11043=PLANE ( 'NONE',  #15049 ) ;
#11046=AXIS2_PLACEMENT_3D ( 'NONE', #22980, #6856, #7110 ) ;
#11054=LINE ( 'NONE', #17772, #20594 ) ;
#11056=ORIENTED_EDGE ( 'NONE', *, *, #11287, .F. ) ;
#11058=PRODUCT_DEFINITION ( 'UNKNOWN', '', #4485, #22059 ) ;
#11063=PLANE ( 'NONE',  #6903 ) ;
#11068=CARTESIAN_POINT ( 'NONE',  ( -0.5000000000000837108, -2.000000000000029310, 7.500000000000007105 ) ) ;
#11074=DIRECTION ( 'NONE',  ( -1.000000000000000000, -1.479114197289387852E-30, 2.013525853228518840E-32 ) ) ;
#11075=VECTOR ( 'NONE', #13635, 1000.000000000000000 ) ;
#11076=CIRCLE ( 'NONE', #2827, 2.550000000000010481 ) ;
#11081=VERTEX_POINT ( 'NONE', #15005 ) ;
#11087=VERTEX_POINT ( 'NONE', #19847 ) ;
#11097=FACE_OUTER_BOUND ( 'NONE', #13650, .T. ) ;
#11102=ADVANCED_FACE ( 'NONE', ( #18085 ), #853, .T. ) ;
#11111=ORIENTED_EDGE ( 'NONE', *, *, #16944, .T. ) ;
#11120=ORIENTED_EDGE ( 'NONE', *, *, #21542, .F. ) ;
#11121=VECTOR ( 'NONE', #10562, 1000.000000000000000 ) ;
#11125=ADVANCED_FACE ( 'NONE', ( #4293 ), #13601, .T. ) ;
#11128=DIRECTION ( 'NONE',  ( -1.000000000000000000, -2.220446049250314067E-16, 5.825996348268307008E-33 ) ) ;
#11132=CARTESIAN_POINT ( 'NONE',  ( -89.70000000000057128, -9.020562075079396891E-14, -2.000000000000001776 ) ) ;
#11134=CARTESIAN_POINT ( 'NONE',  ( -89.70000000000064233, 5.551115123125782702E-14, -2.000000000000001776 ) ) ;
#11135=LINE ( 'NONE', #14788, #7478 ) ;
#11141=CIRCLE ( 'NONE', #19402, 0.5000000000000028866 ) ;
#11143=LINE ( 'NONE', #18326, #1444 ) ;
#11149=DIRECTION ( 'NONE',  ( 0.000000000000000000, 1.000000000000000000, 0.000000000000000000 ) ) ;
#11151=AXIS2_PLACEMENT_3D ( 'NONE', #12189, #17970, #19496 ) ;
#11160=CIRCLE ( 'NONE', #17157, 2.800000000000017142 ) ;
#11161=CARTESIAN_POINT ( 'NONE',  ( -64.00000000000045475, -6.938893903907228378E-14, -2.000000000000001776 ) ) ;
#11167=DIRECTION ( 'NONE',  ( -2.013525853228507892E-32, -6.902532920683810383E-31, 1.000000000000000000 ) ) ;
#11169=DIRECTION ( 'NONE',  ( 1.000000000000000000, 0.000000000000000000, 0.000000000000000000 ) ) ;
#11180=ORIENTED_EDGE ( 'NONE', *, *, #14392, .T. ) ;
#11183=ORIENTED_EDGE ( 'NONE', *, *, #22086, .F. ) ;
#11203=EDGE_CURVE ( 'NONE', #16719, #5817, #11828, .T. ) ;
#11205=ORIENTED_EDGE ( 'NONE', *, *, #19140, .F. ) ;
#11218=CIRCLE ( 'NONE', #11579, 0.5000000000000004441 ) ;
#11227=FACE_OUTER_BOUND ( 'NONE', #14623, .T. ) ;
#11228=EDGE_CURVE ( 'NONE', #9098, #1910, #1242, .T. ) ;
#11233=EDGE_CURVE ( 'NONE', #4291, #6467, #4596, .T. ) ;
#11245=FACE_OUTER_BOUND ( 'NONE', #3361, .T. ) ;
#11256=CARTESIAN_POINT ( 'NONE',  ( -50.65685424949274562, -2.700000000000125855, 8.000000000000062172 ) ) ;
#11260=PLANE ( 'NONE',  #5165 ) ;
#11287=EDGE_CURVE ( 'NONE', #1883, #6815, #4220, .T. ) ;
#11288=ORIENTED_EDGE ( 'NONE', *, *, #21206, .F. ) ;
#11292=DIRECTION ( 'NONE',  ( 1.550910762415566494E-16, 1.000000000000000000, -8.135128085091684243E-31 ) ) ;
#11293=ORIENTED_EDGE ( 'NONE', *, *, #7548, .F. ) ;
#11295=CARTESIAN_POINT ( 'NONE',  ( -2.700000000000119194, -2.000000000000001776, -8.000000000000007105 ) ) ;
#11297=DIRECTION ( 'NONE',  ( -6.938893903907259932E-15, 1.000000000000000000, 1.553069907153866992E-30 ) ) ;
#11316=ORIENTED_EDGE ( 'NONE', *, *, #6078, .F. ) ;
#11317=VERTEX_POINT ( 'NONE', #19583 ) ;
#11329=CARTESIAN_POINT ( 'NONE',  ( -95.20000000000065654, 6.938893903907228378E-15, -2.000000000000001776 ) ) ;
#11331=DIRECTION ( 'NONE',  ( -0.7071067811865532349, 0.7071067811865416886, 1.565905175853764455E-16 ) ) ;
#11333=ORIENTED_EDGE ( 'NONE', *, *, #20656, .F. ) ;
#11346=ORIENTED_EDGE ( 'NONE', *, *, #18713, .T. ) ;
#11350=DIRECTION ( 'NONE',  ( -1.000000000000000000, 2.818925648462279658E-14, 0.000000000000000000 ) ) ;
#11355=ADVANCED_FACE ( 'NONE', ( #6766 ), #11753, .T. ) ;
#11361=AXIS2_PLACEMENT_3D ( 'NONE', #22775, #4533, #789 ) ;
#11372=VECTOR ( 'NONE', #9008, 1000.000000000000000 ) ;
#11378=CIRCLE ( 'NONE', #22274, 0.4999999999999994449 ) ;
#11379=AXIS2_PLACEMENT_3D ( 'NONE', #17551, #13913, #7111 ) ;
#11381=FACE_OUTER_BOUND ( 'NONE', #15821, .T. ) ;
#11386=DIRECTION ( 'NONE',  ( -1.000000000000000000, 1.387778780781436209E-14, -1.404432126150814819E-14 ) ) ;
#11390=EDGE_CURVE ( 'NONE', #9452, #16835, #18064, .T. ) ;
#11392=CARTESIAN_POINT ( 'NONE',  ( -8.326672684688674053E-14, -1.999999999999988010, -7.500000000000034639 ) ) ;
#11394=CARTESIAN_POINT ( 'NONE',  ( -6.000000000000074607, 4.799999999999964295, 7.500000000000062172 ) ) ;
#11402=EDGE_CURVE ( 'NONE', #17530, #13979, #3121, .T. ) ;
#11404=ORIENTED_EDGE ( 'NONE', *, *, #11233, .F. ) ;
#11410=ORIENTED_EDGE ( 'NONE', *, *, #22014, .T. ) ;
#11413=ADVANCED_FACE ( 'NONE', ( #5598 ), #7471, .T. ) ;
#11416=DIRECTION ( 'NONE',  ( 0.7071067811865460184, -0.7071067811865490160, -1.010793663541200360E-16 ) ) ;
#11429=AXIS2_PLACEMENT_3D ( 'NONE', #22514, #2982, #17549 ) ;
#11430=CIRCLE ( 'NONE', #7322, 0.5000000000000029976 ) ;
#11434=ORIENTED_EDGE ( 'NONE', *, *, #12969, .F. ) ;
#11438=CARTESIAN_POINT ( 'NONE',  ( -50.65685424949281668, 0.5000000000000143219, 7.500000000000034639 ) ) ;
#11441=FACE_OUTER_BOUND ( 'NONE', #854, .T. ) ;
#11447=AXIS2_PLACEMENT_3D ( 'NONE', #4955, #10600, #14259 ) ;
#11456=EDGE_CURVE ( 'NONE', #9368, #7127, #8159, .T. ) ;
#11465=EDGE_LOOP ( 'NONE', ( #4138, #9955 ) ) ;
#11479=SURFACE_STYLE_FILL_AREA ( #7618 ) ;
#11480=FACE_OUTER_BOUND ( 'NONE', #11488, .T. ) ;
#11483=AXIS2_PLACEMENT_3D ( 'NONE', #1172, #4806, #4696 ) ;
#11487=ORIENTED_EDGE ( 'NONE', *, *, #3866, .T. ) ;
#11488=EDGE_LOOP ( 'NONE', ( #1768, #2873, #18158, #14828 ) ) ;
#11494=LINE ( 'NONE', #13162, #17897 ) ;
#11495=DIRECTION ( 'NONE',  ( -0.7071067811865456854, -0.7071067811865494601, -1.010793663541192964E-16 ) ) ;
#11510=EDGE_CURVE ( 'NONE', #22149, #21928, #870, .T. ) ;
#11514=CIRCLE ( 'NONE', #11904, 2.000000000000015543 ) ;
#11521=DIRECTION ( 'NONE',  ( -2.013525853228507892E-32, -6.902532920683810383E-31, 1.000000000000000000 ) ) ;
#11522=DIRECTION ( 'NONE',  ( -2.013525853228507892E-32, -6.902532920683810383E-31, 1.000000000000000000 ) ) ;
#11538=DIRECTION ( 'NONE',  ( -2.655250634480531216E-32, 6.902532920683810383E-31, -1.000000000000000000 ) ) ;
#11540=ORIENTED_EDGE ( 'NONE', *, *, #21013, .T. ) ;
#11548=ORIENTED_EDGE ( 'NONE', *, *, #9869, .F. ) ;
#11550=ORIENTED_EDGE ( 'NONE', *, *, #19659, .F. ) ;
#11551=CIRCLE ( 'NONE', #8560, 10.00000000000006395 ) ;
#11554=ADVANCED_FACE ( 'NONE', ( #11565 ), #18749, .T. ) ;
#11556=DIRECTION ( 'NONE',  ( -1.000000000000000000, 1.369518533665891191E-16, 3.560748187531317046E-15 ) ) ;
#11560=CYLINDRICAL_SURFACE ( 'NONE', #13273, 2.550000000000010481 ) ;
#11565=FACE_OUTER_BOUND ( 'NONE', #15309, .T. ) ;
#11567=PRESENTATION_STYLE_ASSIGNMENT (( #16855 ) ) ;
#11574=VERTEX_POINT ( 'NONE', #14035 ) ;
#11577=EDGE_CURVE ( 'NONE', #14890, #16829, #7276, .T. ) ;
#11579=AXIS2_PLACEMENT_3D ( 'NONE', #7391, #15964, #9038 ) ;
#11595=TOROIDAL_SURFACE ( 'NONE', #21016, 5.500000000000000000, 0.5000000000000000000 ) ;
#11607=ORIENTED_EDGE ( 'NONE', *, *, #7124, .F. ) ;
#11617=DIRECTION ( 'NONE',  ( 1.000000000000000000, 0.000000000000000000, 0.000000000000000000 ) ) ;
#11622=EDGE_CURVE ( 'NONE', #10141, #16719, #22296, .T. ) ;
#11629=ORIENTED_EDGE ( 'NONE', *, *, #4829, .F. ) ;
#11633=ORIENTED_EDGE ( 'NONE', *, *, #1458, .T. ) ;
#11642=DIRECTION ( 'NONE',  ( 2.220446049250313081E-16, -1.000000000000000000, 7.025792437124636392E-31 ) ) ;
#11643=ADVANCED_FACE ( 'NONE', ( #10380 ), #15558, .F. ) ;
#11656=ADVANCED_FACE ( 'NONE', ( #8737 ), #12019, .F. ) ;
#11658=ORIENTED_EDGE ( 'NONE', *, *, #1904, .T. ) ;
#11659=ORIENTED_EDGE ( 'NONE', *, *, #7168, .T. ) ;
#11665=CARTESIAN_POINT ( 'NONE',  ( -64.00000000000038369, -3.200000000000088107, -2.000000000000029310 ) ) ;
#11667=EDGE_CURVE ( 'NONE', #19930, #21802, #15512, .T. ) ;
#11679=EDGE_CURVE ( 'NONE', #3004, #17067, #8778, .T. ) ;
#11696=EDGE_CURVE ( 'NONE', #14335, #18914, #14401, .T. ) ;
#11703=DIRECTION ( 'NONE',  ( -1.000000000000000000, 1.577021341797087946E-16, -5.322447028565171744E-15 ) ) ;
#11721=VERTEX_POINT ( 'NONE', #21797 ) ;
#11729=DIRECTION ( 'NONE',  ( -1.000000000000000000, 1.550910762415566494E-16, -8.566929763922626680E-48 ) ) ;
#11737=AXIS2_PLACEMENT_3D ( 'NONE', #21274, #1841, #5392 ) ;
#11738=DIRECTION ( 'NONE',  ( -1.550910762415566494E-16, -1.000000000000000000, 8.135128085091684243E-31 ) ) ;
#11753=TOROIDAL_SURFACE ( 'NONE', #2348, 3.299999999999999822, 0.5000000000000000000 ) ;
#11763=DIRECTION ( 'NONE',  ( -0.7453559924999295649, 0.000000000000000000, 0.6666666666666669627 ) ) ;
#11764=CARTESIAN_POINT ( 'NONE',  ( -95.20000000000065654, -9.714451465470119729E-14, -2.000000000000001776 ) ) ;
#11765=DIRECTION ( 'NONE',  ( 2.013525853228507892E-32, 6.902532920683810383E-31, -1.000000000000000000 ) ) ;
#11766=VECTOR ( 'NONE', #7990, 1000.000000000000000 ) ;
#11771=CARTESIAN_POINT ( 'NONE',  ( -6.000000000000019540, -7.500000000000007105, 7.500000000000062172 ) ) ;
#11773=DIRECTION ( 'NONE',  ( 1.000000000000000000, 0.000000000000000000, 0.000000000000000000 ) ) ;
#11775=DIRECTION ( 'NONE',  ( -1.550910762415566494E-16, -1.000000000000000000, 8.135128085091684243E-31 ) ) ;
#11784=VECTOR ( 'NONE', #21018, 1000.000000000000114 ) ;
#11786=ORIENTED_EDGE ( 'NONE', *, *, #3345, .F. ) ;
#11792=ADVANCED_FACE ( 'NONE', ( #10846 ), #3675, .T. ) ;
#11793=LINE ( 'NONE', #18980, #8489 ) ;
#11804=AXIS2_PLACEMENT_3D ( 'NONE', #8157, #19327, #11905 ) ;
#11805=CIRCLE ( 'NONE', #22716, 10.00000000000006395 ) ;
#11822=EDGE_CURVE ( 'NONE', #6879, #1883, #9081, .T. ) ;
#11823=ADVANCED_FACE ( 'NONE', ( #46 ), #14715, .F. ) ;
#11825=ORIENTED_EDGE ( 'NONE', *, *, #3345, .T. ) ;
#11828=LINE ( 'NONE', #15585, #4987 ) ;
#11832=CARTESIAN_POINT ( 'NONE',  ( -45.01801948466083303, -6.474873734152952309, 8.000000000000062172 ) ) ;
#11833=CARTESIAN_POINT ( 'NONE',  ( -89.70000000000055707, -3.200000000000091660, -1.999999999999946265 ) ) ;
#11834=DIRECTION ( 'NONE',  ( 1.550910762415566494E-16, 1.000000000000000000, -8.135128085091684243E-31 ) ) ;
#11835=DIRECTION ( 'NONE',  ( 0.000000000000000000, 0.000000000000000000, 1.000000000000000000 ) ) ;
#11836=EDGE_CURVE ( 'NONE', #4144, #1136, #6141, .T. ) ;
#11850=LINE ( 'NONE', #2674, #3893 ) ;
#11860=DIRECTION ( 'NONE',  ( -1.000000000000000000, 0.000000000000000000, 0.000000000000000000 ) ) ;
#11865=LINE ( 'NONE', #9875, #20561 ) ;
#11867=CARTESIAN_POINT ( 'NONE',  ( -0.5000000000000975886, 4.799999999999929656, 7.500000000000007105 ) ) ;
#11870=EDGE_LOOP ( 'NONE', ( #6567, #19308, #17328, #15100 ) ) ;
#11877=CARTESIAN_POINT ( 'NONE',  ( -50.65685424949280247, 1.387778780781445676E-14, 8.000000000000090594 ) ) ;
#11886=DIRECTION ( 'NONE',  ( -2.775557561562891351E-14, 1.000000000000000000, 0.000000000000000000 ) ) ;
#11893=ORIENTED_EDGE ( 'NONE', *, *, #5701, .T. ) ;
#11901=DIRECTION ( 'NONE',  ( 2.013525853228507892E-32, 6.902532920683810383E-31, -1.000000000000000000 ) ) ;
#11904=AXIS2_PLACEMENT_3D ( 'NONE', #17676, #6997, #21349 ) ;
#11905=DIRECTION ( 'NONE',  ( 1.000000000000000000, 0.000000000000000000, 0.000000000000000000 ) ) ;
#11906=AXIS2_PLACEMENT_3D ( 'NONE', #4480, #4828, #11998 ) ;
#11908=PLANE ( 'NONE',  #1093 ) ;
#11922=VERTEX_POINT ( 'NONE', #14334 ) ;
#11938=AXIS2_PLACEMENT_3D ( 'NONE', #13464, #6180, #18636 ) ;
#11941=CARTESIAN_POINT ( 'NONE',  ( -50.65685424949267457, -7.632783294297951215E-14, 8.000000000000047962 ) ) ;
#11945=VECTOR ( 'NONE', #13294, 1000.000000000000000 ) ;
#11952=VERTEX_POINT ( 'NONE', #16086 ) ;
#11953=ADVANCED_FACE ( 'NONE', ( #17749 ), #10651, .T. ) ;
#11957=DIRECTION ( 'NONE',  ( -2.013525853228507892E-32, -6.902532920683810383E-31, 1.000000000000000000 ) ) ;
#11959=ORIENTED_EDGE ( 'NONE', *, *, #4211, .T. ) ;
#11961=DIRECTION ( 'NONE',  ( -0.9878135252003128475, 1.532010627492774680E-16, 0.1556420233463030045 ) ) ;
#11969=DIRECTION ( 'NONE',  ( 0.9706398123736367234, 2.735793299299322016E-14, 0.2405376366294291746 ) ) ;
#11975=CARTESIAN_POINT ( 'NONE',  ( -56.91911807125110556, 3.200000000000057021, -8.333333333333358794 ) ) ;
#11981=AXIS2_PLACEMENT_3D ( 'NONE', #21735, #18425, #9377 ) ;
#11985=TOROIDAL_SURFACE ( 'NONE', #20285, 3.500000000000000888, 0.5000000000000000000 ) ;
#11989=ORIENTED_EDGE ( 'NONE', *, *, #7548, .T. ) ;
#11990=DIRECTION ( 'NONE',  ( 2.220446049250313081E-16, -1.000000000000000000, 7.025792437124636392E-31 ) ) ;
#11994=CARTESIAN_POINT ( 'NONE',  ( -43.10883117545714782, -4.565685424949276872, 7.500000000000062172 ) ) ;
#11995=CARTESIAN_POINT ( 'NONE',  ( -55.05572809000125289, -0.5000000000001045830, -10.00000000000006395 ) ) ;
#11998=DIRECTION ( 'NONE',  ( 1.000000000000000000, 2.282530889443153710E-16, 0.000000000000000000 ) ) ;
#12011=ORIENTED_EDGE ( 'NONE', *, *, #17007, .F. ) ;
#12014=CIRCLE ( 'NONE', #4865, 2.500000000000015987 ) ;
#12016=DIRECTION ( 'NONE',  ( -2.220446049250313081E-16, 1.000000000000000000, -7.025792437124636392E-31 ) ) ;
#12019=CYLINDRICAL_SURFACE ( 'NONE', #12138, 2.000000000000015543 ) ;
#12020=DIRECTION ( 'NONE',  ( 1.424116703980815236E-16, 1.000000000000000000, -6.902532920683853297E-31 ) ) ;
#12022=EDGE_CURVE ( 'NONE', #9917, #16719, #10668, .T. ) ;
#12025=DIRECTION ( 'NONE',  ( 1.000000000000000000, 5.328079247643017455E-14, 0.000000000000000000 ) ) ;
#12037=EDGE_CURVE ( 'NONE', #2097, #15576, #11850, .T. ) ;
#12039=DIRECTION ( 'NONE',  ( 0.2405376366294550983, 0.000000000000000000, -0.9706398123736303951 ) ) ;
#12043=DIRECTION ( 'NONE',  ( -1.331202777560457422E-30, -1.000000000000000000, 7.395570986446985676E-31 ) ) ;
#12058=AXIS2_PLACEMENT_3D ( 'NONE', #2334, #9518, #14921 ) ;
#12062=DIRECTION ( 'NONE',  ( -1.000000000000000000, 2.775557561562874627E-14, 0.000000000000000000 ) ) ;
#12074=AXIS2_PLACEMENT_3D ( 'NONE', #10070, #19120, #22896 ) ;
#12086=VERTEX_POINT ( 'NONE', #22684 ) ;
#12093=AXIS2_PLACEMENT_3D ( 'NONE', #15835, #14319, #98 ) ;
#12095=AXIS2_PLACEMENT_3D ( 'NONE', #17362, #11957, #12062 ) ;
#12099=CARTESIAN_POINT ( 'NONE',  ( -64.00000000000045475, 0.5000000000000490719, -1.999999999999974021 ) ) ;
#12106=CARTESIAN_POINT ( 'NONE',  ( -3.200000000000008171, -5.300000000000027356, -8.000000000000007105 ) ) ;
#12109=DIRECTION ( 'NONE',  ( 0.7071067811865535679, 0.7071067811865414665, 0.000000000000000000 ) ) ;
#12120=ADVANCED_FACE ( 'NONE', ( #3495 ), #6675, .T. ) ;
#12121=EDGE_CURVE ( 'NONE', #14335, #21725, #7155, .T. ) ;
#12134=CIRCLE ( 'NONE', #13644, 0.5000000000000019984 ) ;
#12135=CARTESIAN_POINT ( 'NONE',  ( -95.20000000000061391, -9.714451465470119729E-14, 8.000000000000117240 ) ) ;
#12136=TOROIDAL_SURFACE ( 'NONE', #1994, 5.500000000000000000, 0.5000000000000000000 ) ;
#12138=AXIS2_PLACEMENT_3D ( 'NONE', #19556, #10154, #22864 ) ;
#12139=DIRECTION ( 'NONE',  ( 2.013525853228508439E-32, 6.779273404243028164E-31, -1.000000000000000000 ) ) ;
#12144=CARTESIAN_POINT ( 'NONE',  ( -95.20000000000067075, 2.700000000000014833, -1.999999999999974021 ) ) ;
#12151=CIRCLE ( 'NONE', #3519, 6.000000000000037303 ) ;
#12158=ORIENTED_EDGE ( 'NONE', *, *, #23171, .F. ) ;
#12167=DIRECTION ( 'NONE',  ( -2.013525853228507892E-32, -6.902532920683810383E-31, 1.000000000000000000 ) ) ;
#12175=CARTESIAN_POINT ( 'NONE',  ( -43.10883117545713361, 4.565685424949256443, 8.000000000000035527 ) ) ;
#12177=ORIENTED_EDGE ( 'NONE', *, *, #2663, .T. ) ;
#12180=ORIENTED_EDGE ( 'NONE', *, *, #18849, .F. ) ;
#12181=ORIENTED_EDGE ( 'NONE', *, *, #20591, .F. ) ;
#12183=ORIENTED_EDGE ( 'NONE', *, *, #22086, .T. ) ;
#12189=CARTESIAN_POINT ( 'NONE',  ( -42.54314575050785407, -4.000000000000034639, -7.500000000000007105 ) ) ;
#12197=CARTESIAN_POINT ( 'NONE',  ( -65.00000000000052580, 0.5000000000000490719, 3.000000000000002665 ) ) ;
#12213=CARTESIAN_POINT ( 'NONE',  ( -90.63385214007844581, 5.551115123125782702E-14, -7.926881151201908615 ) ) ;
#12214=CARTESIAN_POINT ( 'NONE',  ( -42.54314575050785407, -4.800000000000019362, 8.000000000000007105 ) ) ;
#12217=CARTESIAN_POINT ( 'NONE',  ( -56.54644007500113645, 0.5000000000000143219, -8.666666666666710483 ) ) ;
#12225=FACE_OUTER_BOUND ( 'NONE', #14887, .T. ) ;
#12230=EDGE_CURVE ( 'NONE', #14402, #16051, #1386, .T. ) ;
#12231=ORIENTED_EDGE ( 'NONE', *, *, #9739, .F. ) ;
#12238=CARTESIAN_POINT ( 'NONE',  ( -0.5000000000000559552, -1.999999999999988010, -7.500000000000007105 ) ) ;
#12241=LINE ( 'NONE', #6987, #18426 ) ;
#12252=VECTOR ( 'NONE', #4664, 1000.000000000000000 ) ;
#12256=EDGE_CURVE ( 'NONE', #16051, #9575, #8417, .T. ) ;
#12257=LINE ( 'NONE', #8867, #16765 ) ;
#12265=AXIS2_PLACEMENT_3D ( 'NONE', #2916, #11961, #19144 ) ;
#12267=EDGE_CURVE ( 'NONE', #7689, #9100, #3718, .T. ) ;
#12268=EDGE_LOOP ( 'NONE', ( #12741, #15103, #9473, #17164 ) ) ;
#12269=VECTOR ( 'NONE', #18963, 1000.000000000000000 ) ;
#12279=CARTESIAN_POINT ( 'NONE',  ( -95.20000000000064233, 0.5000000000000073275, 1.000000000000014655 ) ) ;
#12282=FACE_OUTER_BOUND ( 'NONE', #276, .T. ) ;
#12285=CARTESIAN_POINT ( 'NONE',  ( -42.54314575050793934, -5.300000000000020250, 7.500000000000062172 ) ) ;
#12295=ORIENTED_EDGE ( 'NONE', *, *, #7168, .F. ) ;
#12300=VECTOR ( 'NONE', #7677, 1000.000000000000000 ) ;
#12302=ORIENTED_EDGE ( 'NONE', *, *, #12659, .T. ) ;
#12306=TOROIDAL_SURFACE ( 'NONE', #1065, 3.500000000000000888, 0.5000000000000000000 ) ;
#12312=FACE_OUTER_BOUND ( 'NONE', #21114, .T. ) ;
#12317=AXIS2_PLACEMENT_3D ( 'NONE', #6603, #19184, #6720 ) ;
#12319=CARTESIAN_POINT ( 'NONE',  ( -47.82842712474642610, -4.371572875253856516, 8.000000000000076383 ) ) ;
#12323=DIRECTION ( 'NONE',  ( 1.550910762415566494E-16, 1.000000000000000000, -8.135128085091684243E-31 ) ) ;
#12324=DIRECTION ( 'NONE',  ( -1.000000000000000000, -1.479114197289387852E-30, 2.013525853228518840E-32 ) ) ;
#12326=ORIENTED_EDGE ( 'NONE', *, *, #18662, .F. ) ;
#12329=ORIENTED_EDGE ( 'NONE', *, *, #5663, .T. ) ;
#12333=DIRECTION ( 'NONE',  ( 2.220446049250313081E-16, -1.000000000000000000, 7.025792437124636392E-31 ) ) ;
#12338=CARTESIAN_POINT ( 'NONE',  ( -91.02295700146251534, -3.200000000000101874, 6.338518968055054437 ) ) ;
#12339=DIRECTION ( 'NONE',  ( -2.013525853228507892E-32, -6.902532920683810383E-31, 1.000000000000000000 ) ) ;
#12341=DIRECTION ( 'NONE',  ( 1.424116703980815236E-16, 1.000000000000000000, -6.902532920683853297E-31 ) ) ;
#12343=DIRECTION ( 'NONE',  ( 0.1556420233463076119, 0.000000000000000000, 0.9878135252003121813 ) ) ;
#12346=VECTOR ( 'NONE', #4580, 1000.000000000000000 ) ;
#12349=TOROIDAL_SURFACE ( 'NONE', #18761, 9.499999999999998224, 0.5000000000000000000 ) ;
#12350=CIRCLE ( 'NONE', #10481, 2.550000000000010481 ) ;
#12362=FACE_OUTER_BOUND ( 'NONE', #21382, .T. ) ;
#12379=CARTESIAN_POINT ( 'NONE',  ( -55.05572809000125289, -1.179611963664228824E-13, -10.00000000000006395 ) ) ;
#12385=VERTEX_POINT ( 'NONE', #2296 ) ;
#12391=ORIENTED_EDGE ( 'NONE', *, *, #13106, .F. ) ;
#12392=AXIS2_PLACEMENT_3D ( 'NONE', #10064, #2772, #19115 ) ;
#12398=DIRECTION ( 'NONE',  ( 0.000000000000000000, -6.938893903907174735E-15, 1.000000000000000000 ) ) ;
#12407=DIRECTION ( 'NONE',  ( 0.9706398123736299510, 1.232595164407823064E-30, 0.2405376366294566526 ) ) ;
#12416=ORIENTED_EDGE ( 'NONE', *, *, #9869, .T. ) ;
#12419=EDGE_CURVE ( 'NONE', #3579, #5105, #4759, .T. ) ;
#12450=LINE ( 'NONE', #17635, #17096 ) ;
#12454=CYLINDRICAL_SURFACE ( 'NONE', #8018, 0.5000000000000000000 ) ;
#12456=CIRCLE ( 'NONE', #3082, 2.800000000000017586 ) ;
#12459=EDGE_CURVE ( 'NONE', #10770, #17530, #2649, .T. ) ;
#12462=DIRECTION ( 'NONE',  ( 2.013525853228518840E-32, -6.902532920683810383E-31, 1.000000000000000000 ) ) ;
#12465=CARTESIAN_POINT ( 'NONE',  ( -55.05572809000125289, 3.200000000000022382, -10.00000000000006395 ) ) ;
#12477=DIRECTION ( 'NONE',  ( 0.9706398123736370565, 1.133987551255197639E-30, 0.2405376366294281198 ) ) ;
#12478=LINE ( 'NONE', #23101, #13952 ) ;
#12486=VECTOR ( 'NONE', #9460, 1000.000000000000000 ) ;
#12501=VERTEX_POINT ( 'NONE', #10059 ) ;
#12505=ORIENTED_EDGE ( 'NONE', *, *, #1632, .F. ) ;
#12511=ORIENTED_EDGE ( 'NONE', *, *, #19579, .T. ) ;
#12513=DIRECTION ( 'NONE',  ( 2.013525853228507892E-32, 6.902532920683810383E-31, -1.000000000000000000 ) ) ;
#12514=LINE ( 'NONE', #16154, #8756 ) ;
#12516=DIRECTION ( 'NONE',  ( 1.550910762415566494E-16, 1.000000000000000000, -8.135128085091684243E-31 ) ) ;
#12520=EDGE_CURVE ( 'NONE', #15489, #6825, #9939, .T. ) ;
#12523=VECTOR ( 'NONE', #16421, 1000.000000000000000 ) ;
#12534=DIRECTION ( 'NONE',  ( -1.550910762415566494E-16, -1.000000000000000000, 8.135128085091684243E-31 ) ) ;
#12535=EDGE_LOOP ( 'NONE', ( #23261, #22609, #9042, #6095 ) ) ;
#12552=DIRECTION ( 'NONE',  ( -1.000000000000000000, -1.424116703980846297E-16, 1.095779650622964657E-32 ) ) ;
#12559=CARTESIAN_POINT ( 'NONE',  ( -55.25320565519145788, -0.5000000000000281997, 10.00000000000009237 ) ) ;
#12565=VERTEX_POINT ( 'NONE', #7133 ) ;
#12569=ORIENTED_EDGE ( 'NONE', *, *, #10947, .T. ) ;
#12584=CARTESIAN_POINT ( 'NONE',  ( -55.25320565519145788, -2.775557561562891351E-14, 10.00000000000009237 ) ) ;
#12585=DIRECTION ( 'NONE',  ( 2.013525853228507892E-32, 6.902532920683810383E-31, -1.000000000000000000 ) ) ;
#12592=EDGE_CURVE ( 'NONE', #22558, #9917, #22705, .T. ) ;
#12593=VECTOR ( 'NONE', #2587, 1000.000000000000000 ) ;
#12594=ORIENTED_EDGE ( 'NONE', *, *, #17713, .F. ) ;
#12595=ORIENTED_EDGE ( 'NONE', *, *, #4040, .T. ) ;
#12616=ORIENTED_EDGE ( 'NONE', *, *, #15615, .F. ) ;
#12624=ORIENTED_EDGE ( 'NONE', *, *, #13280, .T. ) ;
#12629=DIRECTION ( 'NONE',  ( -1.000000000000000000, 1.424116703980815236E-16, 2.931272055834072749E-32 ) ) ;
#12632=LINE ( 'NONE', #16384, #5640 ) ;
#12636=CARTESIAN_POINT ( 'NONE',  ( -42.54314575050785407, -4.000000000000021316, 8.000000000000007105 ) ) ;
#12640=LINE ( 'NONE', #4353, #10683 ) ;
#12649=VECTOR ( 'NONE', #13227, 1000.000000000000000 ) ;
#12658=FACE_OUTER_BOUND ( 'NONE', #16636, .T. ) ;
#12659=EDGE_CURVE ( 'NONE', #16028, #4291, #5350, .T. ) ;
#12663=DIRECTION ( 'NONE',  ( -1.550910762415566494E-16, -1.000000000000000000, 8.135128085091684243E-31 ) ) ;
#12664=VECTOR ( 'NONE', #12534, 1000.000000000000000 ) ;
#12675=AXIS2_PLACEMENT_3D ( 'NONE', #17674, #14158, #1346 ) ;
#12683=CARTESIAN_POINT ( 'NONE',  ( -65.55642023346354108, 2.700000000000056577, -11.87813525200309783 ) ) ;
#12688=CIRCLE ( 'NONE', #1794, 0.5000000000000029976 ) ;
#12692=DIRECTION ( 'NONE',  ( 1.939787525279694947E-32, -6.902532920683810383E-31, 1.000000000000000000 ) ) ;
#12694=ORIENTED_EDGE ( 'NONE', *, *, #13293, .F. ) ;
#12697=CIRCLE ( 'NONE', #19096, 0.5000000000000029976 ) ;
#12698=ADVANCED_FACE ( 'NONE', ( #10171 ), #17334, .T. ) ;
#12700=CARTESIAN_POINT ( 'NONE',  ( -90.55603112840523750, -6.245004513516505540E-14, -7.432974388601742533 ) ) ;
#12703=EDGE_CURVE ( 'NONE', #6879, #2848, #5470, .T. ) ;
#12705=DIRECTION ( 'NONE',  ( -1.000000000000000000, 0.000000000000000000, 0.000000000000000000 ) ) ;
#12708=( GEOMETRIC_REPRESENTATION_CONTEXT ( 3 ) GLOBAL_UNCERTAINTY_ASSIGNED_CONTEXT ( ( #18049 ) ) GLOBAL_UNIT_ASSIGNED_CONTEXT ( ( #441, #9615, #7193 ) ) REPRESENTATION_CONTEXT ( 'NONE', 'WORKASPACE' ) );
#12725=CARTESIAN_POINT ( 'NONE',  ( -43.46238456605043865, -4.919238815542549936, 7.500000000000062172 ) ) ;
#12741=ORIENTED_EDGE ( 'NONE', *, *, #22197, .T. ) ;
#12744=ORIENTED_EDGE ( 'NONE', *, *, #21171, .F. ) ;
#12748=ORIENTED_EDGE ( 'NONE', *, *, #3551, .T. ) ;
#12750=ADVANCED_FACE ( 'NONE', ( #21704 ), #2154, .F. ) ;
#12751=DIRECTION ( 'NONE',  ( 2.013525853228507892E-32, 6.902532920683810383E-31, -1.000000000000000000 ) ) ;
#12755=CARTESIAN_POINT ( 'NONE',  ( -45.56568542494964191, 2.108831175456939100, -8.000000000000062172 ) ) ;
#12757=CARTESIAN_POINT ( 'NONE',  ( -90.55603112840530855, 3.200000000000057021, -7.432974388601742533 ) ) ;
#12758=CARTESIAN_POINT ( 'NONE',  ( -45.01801948466087566, -6.474873734152949645, 7.500000000000089706 ) ) ;
#12762=ADVANCED_FACE ( 'NONE', ( #7236 ), #10751, .F. ) ;
#12767=DIRECTION ( 'NONE',  ( 2.220446049250313081E-16, -1.000000000000000000, 7.025792437124636392E-31 ) ) ;
#12768=CIRCLE ( 'NONE', #15011, 10.00000000000006395 ) ;
#12769=ORIENTED_EDGE ( 'NONE', *, *, #20475, .F. ) ;
#12772=EDGE_CURVE ( 'NONE', #21928, #2848, #4035, .T. ) ;
#12779=CYLINDRICAL_SURFACE ( 'NONE', #21143, 2.550000000000010481 ) ;
#12791=PLANE ( 'NONE',  #2580 ) ;
#12792=FACE_OUTER_BOUND ( 'NONE', #15475, .T. ) ;
#12797=CARTESIAN_POINT ( 'NONE',  ( -55.05572809000118184, -2.700000000000125855, -8.000000000000062172 ) ) ;
#12807=ORIENTED_EDGE ( 'NONE', *, *, #15099, .F. ) ;
#12808=DIRECTION ( 'NONE',  ( -1.000000000000000000, 0.000000000000000000, 0.000000000000000000 ) ) ;
#12814=AXIS2_PLACEMENT_3D ( 'NONE', #21489, #23257, #7020 ) ;
#12823=ORIENTED_EDGE ( 'NONE', *, *, #18533, .T. ) ;
#12840=CARTESIAN_POINT ( 'NONE',  ( -50.65685424949267457, -7.200000000000049916, 8.000000000000035527 ) ) ;
#12845=PLANE ( 'NONE',  #21304 ) ;
#12854=ORIENTED_EDGE ( 'NONE', *, *, #18762, .F. ) ;
#12861=AXIS2_PLACEMENT_3D ( 'NONE', #535, #16740, #18752 ) ;
#12865=ORIENTED_EDGE ( 'NONE', *, *, #13179, .F. ) ;
#12871=DIRECTION ( 'NONE',  ( 1.550910762415566494E-16, 1.000000000000000000, -8.135128085091684243E-31 ) ) ;
#12873=LINE ( 'NONE', #18746, #12486 ) ;
#12885=EDGE_LOOP ( 'NONE', ( #5721, #8997, #19923, #9244 ) ) ;
#12887=AXIS2_PLACEMENT_3D ( 'NONE', #18397, #19939, #1816 ) ;
#12896=DIRECTION ( 'NONE',  ( -2.013525853228507892E-32, -6.902532920683810383E-31, 1.000000000000000000 ) ) ;
#12903=CARTESIAN_POINT ( 'NONE',  ( -43.46238456605041023, -4.919238815542515297, -7.500000000000007105 ) ) ;
#12905=TOROIDAL_SURFACE ( 'NONE', #19675, 5.500000000000003553, 0.5000000000000000000 ) ;
#12914=DIRECTION ( 'NONE',  ( 2.013525853228507892E-32, 6.902532920683810383E-31, -1.000000000000000000 ) ) ;
#12921=CARTESIAN_POINT ( 'NONE',  ( -45.01801948466074776, -6.474873734152911453, -7.500000000000034639 ) ) ;
#12926=DIRECTION ( 'NONE',  ( 0.7071067811865490160, 0.7071067811865460184, 1.565905175853766674E-16 ) ) ;
#12938=DIRECTION ( 'NONE',  ( 0.7071067811865485719, -0.7071067811865464625, -1.010793663541191485E-16 ) ) ;
#12939=DIRECTION ( 'NONE',  ( -2.013525853228507892E-32, -6.902532920683810383E-31, 1.000000000000000000 ) ) ;
#12947=CIRCLE ( 'NONE', #22727, 2.000000000000015543 ) ;
#12953=EDGE_CURVE ( 'NONE', #12086, #3004, #21179, .T. ) ;
#12955=EDGE_LOOP ( 'NONE', ( #20888, #10485, #22885, #2945 ) ) ;
#12969=EDGE_CURVE ( 'NONE', #15940, #11081, #13279, .T. ) ;
#12978=ORIENTED_EDGE ( 'NONE', *, *, #2102, .F. ) ;
#12982=ORIENTED_EDGE ( 'NONE', *, *, #23086, .T. ) ;
#12989=CARTESIAN_POINT ( 'NONE',  ( -42.54314575050782565, -4.000000000000034639, -8.000000000000007105 ) ) ;
#12991=DIRECTION ( 'NONE',  ( -1.000000000000000000, 1.550910762415566494E-16, 1.495339968488870838E-47 ) ) ;
#13004=EDGE_CURVE ( 'NONE', #7574, #22801, #5728, .T. ) ;
#13014=ORIENTED_EDGE ( 'NONE', *, *, #1771, .F. ) ;
#13018=LINE ( 'NONE', #6311, #17356 ) ;
#13019=CYLINDRICAL_SURFACE ( 'NONE', #16590, 0.8000000000000090372 ) ;
#13025=CARTESIAN_POINT ( 'NONE',  ( -6.000000000000143885, -2.000000000000043521, -8.000000000000035527 ) ) ;
#13027=CARTESIAN_POINT ( 'NONE',  ( -56.54644007500113645, 2.700000000000056577, -8.666666666666710483 ) ) ;
#13030=TOROIDAL_SURFACE ( 'NONE', #3630, 3.299999999999999822, 0.5000000000000000000 ) ;
#13040=DIRECTION ( 'NONE',  ( 1.000000000000000000, 2.365532012695626003E-16, 8.673617379883962502E-16 ) ) ;
#13044=AXIS2_PLACEMENT_3D ( 'NONE', #12465, #14477, #18117 ) ;
#13045=DIRECTION ( 'NONE',  ( -0.9878135252003128475, -2.193386639427060968E-16, 0.1556420233463030045 ) ) ;
#13047=CARTESIAN_POINT ( 'NONE',  ( -65.00000000000046896, -6.938893903907228378E-14, 3.000000000000030198 ) ) ;
#13051=CIRCLE ( 'NONE', #17537, 2.000000000000015543 ) ;
#13056=EDGE_CURVE ( 'NONE', #12086, #22937, #2393, .T. ) ;
#13059=TOROIDAL_SURFACE ( 'NONE', #19071, 5.500000000000003553, 0.5000000000000000000 ) ;
#13066=ORIENTED_EDGE ( 'NONE', *, *, #184, .T. ) ;
#13067=DIRECTION ( 'NONE',  ( -1.734723475976796642E-15, 0.000000000000000000, -1.000000000000000000 ) ) ;
#13068=AXIS2_PLACEMENT_3D ( 'NONE', #17207, #4744, #18866 ) ;
#13070=DIRECTION ( 'NONE',  ( -1.000000000000000000, -1.144237745222090235E-17, -2.013525853228508713E-32 ) ) ;
#13073=DIRECTION ( 'NONE',  ( 0.9706398123736300620, -2.860973184834435137E-14, 0.2405376366294562085 ) ) ;
#13077=CARTESIAN_POINT ( 'NONE',  ( -6.000000000000088818, 7.999999999999958256, 8.000000000000035527 ) ) ;
#13083=FACE_OUTER_BOUND ( 'NONE', #4635, .T. ) ;
#13084=CARTESIAN_POINT ( 'NONE',  ( -66.55000000000046612, 6.188383139260622304E-14, -1.999999999999974021 ) ) ;
#13088=VERTEX_POINT ( 'NONE', #7544 ) ;
#13093=EDGE_LOOP ( 'NONE', ( #8900, #11316, #11056, #17508 ) ) ;
#13104=PLANE ( 'NONE',  #14026 ) ;
#13105=CARTESIAN_POINT ( 'NONE',  ( -65.00000000000052580, 5.551115123125782702E-14, 3.000000000000002665 ) ) ;
#13106=EDGE_CURVE ( 'NONE', #3579, #9134, #17390, .T. ) ;
#13109=CARTESIAN_POINT ( 'NONE',  ( -91.14322581977734217, 2.700000000000014833, 6.823838874241886288 ) ) ;
#13124=AXIS2_PLACEMENT_3D ( 'NONE', #16411, #5856, #15006 ) ;
#13129=ORIENTED_EDGE ( 'NONE', *, *, #943, .T. ) ;
#13137=ADVANCED_FACE ( 'NONE', ( #2588 ), #487, .T. ) ;
#13144=DIRECTION ( 'NONE',  ( 1.331202777560457422E-30, 1.000000000000000000, -7.395570986446985676E-31 ) ) ;
#13150=FILL_AREA_STYLE_COLOUR ( '', #4433 ) ;
#13154=ORIENTED_EDGE ( 'NONE', *, *, #1182, .F. ) ;
#13159=ORIENTED_EDGE ( 'NONE', *, *, #14695, .T. ) ;
#13162=CARTESIAN_POINT ( 'NONE',  ( -56.87767137932630845, -4.163336342344337027E-14, 8.833333333333401427 ) ) ;
#13163=CARTESIAN_POINT ( 'NONE',  ( -51.07487373415331433, 0.4180194846605325698, 7.500000000000062172 ) ) ;
#13171=LINE ( 'NONE', #2105, #21232 ) ;
#13172=DIRECTION ( 'NONE',  ( 2.013525853228507892E-32, 6.902532920683810383E-31, -1.000000000000000000 ) ) ;
#13177=AXIS2_PLACEMENT_3D ( 'NONE', #7549, #2123, #14605 ) ;
#13179=EDGE_CURVE ( 'NONE', #21802, #20271, #8702, .T. ) ;
#13184=CARTESIAN_POINT ( 'NONE',  ( -42.54314575050782565, -5.300000000000037126, -8.000000000000007105 ) ) ;
#13190=PLANE ( 'NONE',  #21905 ) ;
#13194=DIRECTION ( 'NONE',  ( 1.000000000000000000, 1.424116703980846297E-16, -1.095779650622964657E-32 ) ) ;
#13198=CARTESIAN_POINT ( 'NONE',  ( -65.55642023346354108, 6.245004513516505540E-14, -11.87813525200309783 ) ) ;
#13200=CIRCLE ( 'NONE', #16195, 0.5000000000000029976 ) ;
#13214=FACE_OUTER_BOUND ( 'NONE', #21719, .T. ) ;
#13218=CARTESIAN_POINT ( 'NONE',  ( -57.28378781035998912, -2.775557561562891351E-14, 8.541666666666767327 ) ) ;
#13222=CYLINDRICAL_SURFACE ( 'NONE', #12861, 6.000000000000047073 ) ;
#13227=DIRECTION ( 'NONE',  ( 2.013525853228507892E-32, 6.902532920683810383E-31, -1.000000000000000000 ) ) ;
#13236=ORIENTED_EDGE ( 'NONE', *, *, #19427, .T. ) ;
#13239=ORIENTED_EDGE ( 'NONE', *, *, #4318, .F. ) ;
#13242=ORIENTED_EDGE ( 'NONE', *, *, #23047, .T. ) ;
#13252=DIRECTION ( 'NONE',  ( -0.7071067811865507924, -0.7071067811865441310, -2.121016688166342479E-16 ) ) ;
#13257=AXIS2_PLACEMENT_3D ( 'NONE', #12758, #19943, #14640 ) ;
#13272=DIRECTION ( 'NONE',  ( -0.1556420233463035319, 1.944076074078271124E-17, -0.9878135252003127365 ) ) ;
#13273=AXIS2_PLACEMENT_3D ( 'NONE', #1414, #15756, #2627 ) ;
#13279=CIRCLE ( 'NONE', #11016, 0.5000000000000029976 ) ;
#13280=EDGE_CURVE ( 'NONE', #22801, #2139, #6594, .T. ) ;
#13286=CARTESIAN_POINT ( 'NONE',  ( -43.10883117545717624, 5.299999999999998934, 8.000000000000076383 ) ) ;
#13287=DIRECTION ( 'NONE',  ( 1.000000000000000000, -2.785515554063903297E-14, -1.815210279346915817E-30 ) ) ;
#13290=ADVANCED_FACE ( 'NONE', ( #22827 ), #11985, .T. ) ;
#13293=EDGE_CURVE ( 'NONE', #21240, #7622, #2604, .T. ) ;
#13294=DIRECTION ( 'NONE',  ( 1.000000000000000000, 2.220446049250314067E-16, -5.825996348268307008E-33 ) ) ;
#13305=DIRECTION ( 'NONE',  ( 0.000000000000000000, 0.000000000000000000, -1.000000000000000000 ) ) ;
#13306=AXIS2_PLACEMENT_3D ( 'NONE', #2860, #14496, #16238 ) ;
#13321=LINE ( 'NONE', #15301, #19475 ) ;
#13333=ORIENTED_EDGE ( 'NONE', *, *, #10402, .F. ) ;
#13338=CARTESIAN_POINT ( 'NONE',  ( -50.65685424949275983, 2.700000000000021938, 7.500000000000062172 ) ) ;
#13342=CIRCLE ( 'NONE', #6207, 0.5000000000000028866 ) ;
#13344=DIRECTION ( 'NONE',  ( -0.2405376366294420254, 0.000000000000000000, 0.9706398123736336148 ) ) ;
#13351=ORIENTED_EDGE ( 'NONE', *, *, #12953, .T. ) ;
#13356=ORIENTED_EDGE ( 'NONE', *, *, #3938, .T. ) ;
#13359=VECTOR ( 'NONE', #3415, 1000.000000000000000 ) ;
#13360=ORIENTED_EDGE ( 'NONE', *, *, #20074, .T. ) ;
#13364=DIRECTION ( 'NONE',  ( 2.013525853228507892E-32, 6.902532920683810383E-31, -1.000000000000000000 ) ) ;
#13372=PLANE ( 'NONE',  #4831 ) ;
#13378=VERTEX_POINT ( 'NONE', #122 ) ;
#13383=ADVANCED_FACE ( 'NONE', ( #9283 ), #18105, .T. ) ;
#13395=DIRECTION ( 'NONE',  ( 2.013525853228507892E-32, 6.902532920683810383E-31, -1.000000000000000000 ) ) ;
#13398=CARTESIAN_POINT ( 'NONE',  ( -42.54314575050793934, 3.999999999999996447, 7.500000000000062172 ) ) ;
#13400=DIRECTION ( 'NONE',  ( -1.000000000000000000, -1.479114197289388027E-30, -2.013525853228507892E-32 ) ) ;
#13415=EDGE_CURVE ( 'NONE', #15826, #18197, #8256, .T. ) ;
#13416=DIRECTION ( 'NONE',  ( 1.000000000000000000, 0.000000000000000000, 0.000000000000000000 ) ) ;
#13436=DIRECTION ( 'NONE',  ( 2.081668171172155892E-14, 0.000000000000000000, 1.000000000000000000 ) ) ;
#13440=EDGE_LOOP ( 'NONE', ( #3269, #5006, #17243, #5014 ) ) ;
#13445=ORIENTED_EDGE ( 'NONE', *, *, #19004, .F. ) ;
#13449=CIRCLE ( 'NONE', #10822, 10.00000000000006395 ) ;
#13450=DIRECTION ( 'NONE',  ( 0.000000000000000000, 0.000000000000000000, -1.000000000000000000 ) ) ;
#13453=CYLINDRICAL_SURFACE ( 'NONE', #3992, 0.5000000000000000000 ) ;
#13454=FACE_OUTER_BOUND ( 'NONE', #9882, .T. ) ;
#13464=CARTESIAN_POINT ( 'NONE',  ( -55.25320565519145788, 3.200000000000098765, 10.00000000000009237 ) ) ;
#13482=ORIENTED_EDGE ( 'NONE', *, *, #19301, .T. ) ;
#13494=DIRECTION ( 'NONE',  ( 2.013525853228508439E-32, 6.779273404243028164E-31, -1.000000000000000000 ) ) ;
#13498=DIRECTION ( 'NONE',  ( 1.000000000000000000, -1.389842848855773151E-62, 2.013525853228507618E-32 ) ) ;
#13499=ORIENTED_EDGE ( 'NONE', *, *, #1458, .F. ) ;
#13501=ORIENTED_EDGE ( 'NONE', *, *, #21542, .T. ) ;
#13503=ORIENTED_EDGE ( 'NONE', *, *, #22174, .F. ) ;
#13505=CIRCLE ( 'NONE', #2233, 0.5000000000000029976 ) ;
#13509=CARTESIAN_POINT ( 'NONE',  ( -50.65685424949280247, 0.5000000000000213163, 8.000000000000090594 ) ) ;
#13510=DIRECTION ( 'NONE',  ( 0.7071067811865554553, -0.7071067811865398012, 0.000000000000000000 ) ) ;
#13511=DIRECTION ( 'NONE',  ( -2.013525853228507892E-32, -6.902532920683810383E-31, 1.000000000000000000 ) ) ;
#13519=DIRECTION ( 'NONE',  ( -1.550910762415566494E-16, -1.000000000000000000, 8.135128085091684243E-31 ) ) ;
#13520=ORIENTED_EDGE ( 'NONE', *, *, #19999, .T. ) ;
#13532=EDGE_CURVE ( 'NONE', #1694, #18669, #19132, .T. ) ;
#13533=FACE_OUTER_BOUND ( 'NONE', #12955, .T. ) ;
#13536=VERTEX_POINT ( 'NONE', #6650 ) ;
#13538=DIRECTION ( 'NONE',  ( -1.000000000000000000, -1.424116703980846297E-16, 1.095779650622964657E-32 ) ) ;
#13546=CARTESIAN_POINT ( 'NONE',  ( -44.61801948466079182, -6.874873734152946447, -7.500000000000007105 ) ) ;
#13550=PLANE ( 'NONE',  #16831 ) ;
#13553=ADVANCED_FACE ( 'NONE', ( #455 ), #7634, .T. ) ;
#13561=AXIS2_PLACEMENT_3D ( 'NONE', #16698, #607, #9547 ) ;
#13567=EDGE_CURVE ( 'NONE', #16331, #11922, #12014, .T. ) ;
#13581=EDGE_CURVE ( 'NONE', #17067, #22937, #12768, .T. ) ;
#13592=ORIENTED_EDGE ( 'NONE', *, *, #17002, .F. ) ;
#13595=AXIS2_PLACEMENT_3D ( 'NONE', #12921, #15021, #14564 ) ;
#13601=PLANE ( 'NONE',  #9112 ) ;
#13607=DIRECTION ( 'NONE',  ( -1.000000000000000000, 1.445602896647327823E-16, 0.000000000000000000 ) ) ;
#13616=ADVANCED_FACE ( 'NONE', ( #17826 ), #15921, .T. ) ;
#13618=ORIENTED_EDGE ( 'NONE', *, *, #21482, .T. ) ;
#13624=CYLINDRICAL_SURFACE ( 'NONE', #21201, 0.5000000000000004441 ) ;
#13627=ORIENTED_EDGE ( 'NONE', *, *, #13567, .F. ) ;
#13635=DIRECTION ( 'NONE',  ( 1.000000000000000000, 1.424116703980846297E-16, -1.095779650622964657E-32 ) ) ;
#13637=DIRECTION ( 'NONE',  ( -1.000000000000000000, 1.734723475976796001E-16, 0.000000000000000000 ) ) ;
#13639=DIRECTION ( 'NONE',  ( -1.387778780781445676E-14, -1.000000000000000000, 0.000000000000000000 ) ) ;
#13644=AXIS2_PLACEMENT_3D ( 'NONE', #4583, #2704, #11763 ) ;
#13650=EDGE_LOOP ( 'NONE', ( #1803, #5578, #18023, #21838 ) ) ;
#13652=LINE ( 'NONE', #11877, #10713 ) ;
#13658=CARTESIAN_POINT ( 'NONE',  ( -92.25000000000066791, 3.200000000000056577, -2.000000000000001776 ) ) ;
#13670=EDGE_LOOP ( 'NONE', ( #22183, #22890, #18587, #20154 ) ) ;
#13692=EDGE_CURVE ( 'NONE', #6467, #15165, #19468, .T. ) ;
#13695=EDGE_CURVE ( 'NONE', #5105, #11001, #14286, .T. ) ;
#13706=ORIENTED_EDGE ( 'NONE', *, *, #16417, .F. ) ;
#13707=ADVANCED_FACE ( 'NONE', ( #11097 ), #7353, .T. ) ;
#13714=ORIENTED_EDGE ( 'NONE', *, *, #16456, .T. ) ;
#13717=ADVANCED_FACE ( 'NONE', ( #185 ), #3016, .T. ) ;
#13718=DIRECTION ( 'NONE',  ( -2.013525853228507892E-32, -6.902532920683810383E-31, 1.000000000000000000 ) ) ;
#13723=CARTESIAN_POINT ( 'NONE',  ( -45.91923881554277642, 2.462384566050156209, 7.500000000000047962 ) ) ;
#13728=CIRCLE ( 'NONE', #5074, 6.000000000000047073 ) ;
#13740=AXIS2_PLACEMENT_3D ( 'NONE', #5396, #19850, #16414 ) ;
#13748=EDGE_CURVE ( 'NONE', #19870, #8087, #12632, .T. ) ;
#13752=LINE ( 'NONE', #1057, #671 ) ;
#13757=CARTESIAN_POINT ( 'NONE',  ( -67.40537636629490237, -1.249000902703301108E-13, 12.70639812373640432 ) ) ;
#13768=CARTESIAN_POINT ( 'NONE',  ( -43.06238456605038323, -5.319238815542544074, -8.000000000000007105 ) ) ;
#13773=ADVANCED_FACE ( 'NONE', ( #2397 ), #10868, .T. ) ;
#13779=AXIS2_PLACEMENT_3D ( 'NONE', #21037, #2563, #11729 ) ;
#13780=CARTESIAN_POINT ( 'NONE',  ( -42.54314575050795355, 5.299999999999991829, -7.500000000000007105 ) ) ;
#13782=VECTOR ( 'NONE', #20532, 1000.000000000000000 ) ;
#13789=ORIENTED_EDGE ( 'NONE', *, *, #8005, .T. ) ;
#13791=DIRECTION ( 'NONE',  ( 0.000000000000000000, 0.000000000000000000, -1.000000000000000000 ) ) ;
#13795=LINE ( 'NONE', #10605, #2642 ) ;
#13804=TOROIDAL_SURFACE ( 'NONE', #8165, 9.499999999999998224, 0.5000000000000000000 ) ;
#13805=DIRECTION ( 'NONE',  ( 1.000000000000000000, 2.220446049250313081E-16, -3.656342123407104498E-48 ) ) ;
#13808=PRODUCT ( 'Hold Down Arm', 'Hold Down Arm', '', ( #369 ) ) ;
#13809=ORIENTED_EDGE ( 'NONE', *, *, #1471, .F. ) ;
#13815=ORIENTED_EDGE ( 'NONE', *, *, #7092, .T. ) ;
#13816=EDGE_CURVE ( 'NONE', #16719, #18130, #5707, .T. ) ;
#13817=ORIENTED_EDGE ( 'NONE', *, *, #18878, .T. ) ;
#13820=EDGE_CURVE ( 'NONE', #16720, #6492, #3926, .T. ) ;
#13824=CARTESIAN_POINT ( 'NONE',  ( -2.700000000000091216, 1.999999999999911626, 7.500000000000034639 ) ) ;
#13830=DIRECTION ( 'NONE',  ( -1.000000000000000000, 1.365024226554777796E-62, -2.013525853228508439E-32 ) ) ;
#13833=ADVANCED_FACE ( 'NONE', ( #529 ), #22549, .T. ) ;
#13838=EDGE_CURVE ( 'NONE', #22909, #9299, #2044, .T. ) ;
#13847=ORIENTED_EDGE ( 'NONE', *, *, #17007, .T. ) ;
#13863=EDGE_CURVE ( 'NONE', #17750, #7689, #10149, .T. ) ;
#13868=DIRECTION ( 'NONE',  ( -1.331202777560457422E-30, -1.000000000000000000, 7.395570986446985676E-31 ) ) ;
#13869=EDGE_LOOP ( 'NONE', ( #19137, #20507, #7093, #10363 ) ) ;
#13870=EDGE_CURVE ( 'NONE', #2421, #16051, #9926, .T. ) ;
#13871=TOROIDAL_SURFACE ( 'NONE', #5985, 2.500000000000003997, 0.5000000000000000000 ) ;
#13876=VERTEX_POINT ( 'NONE', #2980 ) ;
#13877=AXIS2_PLACEMENT_3D ( 'NONE', #1249, #4650, #8186 ) ;
#13883=ORIENTED_EDGE ( 'NONE', *, *, #18439, .F. ) ;
#13891=CARTESIAN_POINT ( 'NONE',  ( -42.54314575050782565, -4.000000000000034639, -8.000000000000007105 ) ) ;
#13913=DIRECTION ( 'NONE',  ( 0.5833333333333275972, 1.380506584136762077E-30, -0.8122328620674178490 ) ) ;
#13916=FACE_OUTER_BOUND ( 'NONE', #10277, .T. ) ;
#13919=DIRECTION ( 'NONE',  ( 1.000000000000000000, -1.550910762415513985E-16, -3.012982189080959477E-32 ) ) ;
#13948=VERTEX_POINT ( 'NONE', #10036 ) ;
#13949=EDGE_LOOP ( 'NONE', ( #15188, #16747, #16833, #21269 ) ) ;
#13952=VECTOR ( 'NONE', #10603, 1000.000000000000114 ) ;
#13953=ORIENTED_EDGE ( 'NONE', *, *, #5098, .F. ) ;
#13964=CARTESIAN_POINT ( 'NONE',  ( -9.714451465470119729E-14, 1.999999999999932498, -7.500000000000062172 ) ) ;
#13976=DIRECTION ( 'NONE',  ( -1.000000000000000000, 1.550910762415513985E-16, 3.012982189080959477E-32 ) ) ;
#13979=VERTEX_POINT ( 'NONE', #22275 ) ;
#13982=ADVANCED_FACE ( 'NONE', ( #13454 ), #5284, .T. ) ;
#13984=VERTEX_POINT ( 'NONE', #3333 ) ;
#13987=AXIS2_PLACEMENT_3D ( 'NONE', #1338, #12139, #22396 ) ;
#13990=ORIENTED_EDGE ( 'NONE', *, *, #22199, .F. ) ;
#13992=DIRECTION ( 'NONE',  ( 1.550910762415566494E-16, 1.000000000000000000, -8.135128085091684243E-31 ) ) ;
#13994=EDGE_LOOP ( 'NONE', ( #13014, #19005, #15801, #12624 ) ) ;
#13996=LINE ( 'NONE', #6368, #15354 ) ;
#13997=EDGE_CURVE ( 'NONE', #5668, #9452, #13795, .T. ) ;
#14002=EDGE_CURVE ( 'NONE', #14457, #17272, #12241, .T. ) ;
#14007=ADVANCED_FACE ( 'NONE', ( #14264 ), #1519, .T. ) ;
#14018=ORIENTED_EDGE ( 'NONE', *, *, #12703, .T. ) ;
#14026=AXIS2_PLACEMENT_3D ( 'NONE', #19289, #19175, #7808 ) ;
#14027=EDGE_CURVE ( 'NONE', #6998, #13536, #3407, .T. ) ;
#14034=LINE ( 'NONE', #23221, #17829 ) ;
#14035=CARTESIAN_POINT ( 'NONE',  ( -55.05572809000119605, -3.200000000000088107, -7.500000000000062172 ) ) ;
#14036=DIRECTION ( 'NONE',  ( 1.550910762415566494E-16, 1.000000000000000000, -8.135128085091684243E-31 ) ) ;
#14037=DIRECTION ( 'NONE',  ( -1.000000000000000000, 1.550910762415566494E-16, -2.686847401719668638E-48 ) ) ;
#14043=EDGE_LOOP ( 'NONE', ( #21005, #12769, #658, #12295 ) ) ;
#14046=ORIENTED_EDGE ( 'NONE', *, *, #14900, .T. ) ;
#14055=DIRECTION ( 'NONE',  ( 1.000000000000000000, 2.385244779468082934E-14, 0.000000000000000000 ) ) ;
#14061=CLOSED_SHELL ( 'NONE', ( #8829, #11643, #9117, #17588, #9380, #18728, #10350, #8953, #14575, #3715, #1318, #9791, #9549, #4743, #4408, #5894, #14738, #4519, #5240, #1767, #4840, #6862, #11017, #13383, #21390, #3055, #8297, #11792, #19309, #16180, #2650, #3799, #11823, #23137, #15431, #3207, #8365, #12762, #10982, #17305, #7711, #17963, #1616, #11125, #7505, #14844, #17123, #4541, #3200, #19608, #9400, #4487, #22414, #19863, #19841, #7499, #11554, #16982, #18589, #20721, #22341, #13616, #12750, #8937, #14078, #15137, #13707, #11656, #2351, #5223, #9999, #13553, #10378, #6972, #6968, #7578, #3782, #13773, #7788, #549, #13137, #11102, #17381, #5649, #16296, #7487, #21149, #4604, #19592, #15707, #8407, #14865, #4610, #8140, #7919, #16530, #6415, #19595, #18602, #7382, #22678, #18434, #2267, #13717, #17206, #7945, #3052, #21630, #7883, #22488, #2482, #11413, #1313, #13290, #11953, #15680, #16239, #8134, #3653, #7227, #14137, #10446, #11355, #12698, #6513, #1180, #19368, #22078, #4918, #14007, #9691, #15906, #3024, #18356, #13982, #13833, #10399, #1123, #15269, #10740, #10325, #6378, #10684, #10510, #2468, #14426, #5807, #5311, #22453, #1059, #12120, #22158, #6478, #10697, #19629, #101, #21915, #10252, #6814, #9533, #2529, #21792, #4577, #3768, #10829, #15242 ) ) ;
#14069=DIRECTION ( 'NONE',  ( 0.000000000000000000, 0.000000000000000000, -1.000000000000000000 ) ) ;
#14070=FACE_OUTER_BOUND ( 'NONE', #8316, .T. ) ;
#14073=EDGE_LOOP ( 'NONE', ( #17249, #15647, #21262, #3086 ) ) ;
#14078=ADVANCED_FACE ( 'NONE', ( #10376 ), #15554, .T. ) ;
#14079=ORIENTED_EDGE ( 'NONE', *, *, #4167, .T. ) ;
#14080=EDGE_LOOP ( 'NONE', ( #13129, #6186, #5791, #3939 ) ) ;
#14084=CARTESIAN_POINT ( 'NONE',  ( -6.000000000000102141, 4.799999999999964295, 8.000000000000047962 ) ) ;
#14105=EDGE_LOOP ( 'NONE', ( #16598, #8755, #6677, #11548 ) ) ;
#14110=CARTESIAN_POINT ( 'NONE',  ( -64.00000000000045475, 4.857225732735059864E-14, -1.999999999999974021 ) ) ;
#14114=DIRECTION ( 'NONE',  ( 2.013525853228507892E-32, 6.902532920683810383E-31, -1.000000000000000000 ) ) ;
#14129=ORIENTED_EDGE ( 'NONE', *, *, #10223, .T. ) ;
#14132=ORIENTED_EDGE ( 'NONE', *, *, #20728, .F. ) ;
#14134=AXIS2_PLACEMENT_3D ( 'NONE', #17031, #15621, #4453 ) ;
#14136=ORIENTED_EDGE ( 'NONE', *, *, #20885, .T. ) ;
#14137=ADVANCED_FACE ( 'NONE', ( #257 ), #21567, .T. ) ;
#14150=DIRECTION ( 'NONE',  ( -2.013525853228507892E-32, -6.902532920683810383E-31, 1.000000000000000000 ) ) ;
#14155=DIRECTION ( 'NONE',  ( 1.000000000000000000, 0.000000000000000000, 0.000000000000000000 ) ) ;
#14157=AXIS2_PLACEMENT_3D ( 'NONE', #14644, #14183, #16390 ) ;
#14158=DIRECTION ( 'NONE',  ( -1.331202777560457422E-30, -1.000000000000000000, 7.395570986446985676E-31 ) ) ;
#14172=AXIS2_PLACEMENT_3D ( 'NONE', #13891, #1422, #11773 ) ;
#14173=AXIS2_PLACEMENT_3D ( 'NONE', #4007, #16474, #2125 ) ;
#14183=DIRECTION ( 'NONE',  ( -0.6666666666666649643, -4.683861624749726065E-31, -0.7453559924999314523 ) ) ;
#14189=CIRCLE ( 'NONE', #22080, 2.500000000000015987 ) ;
#14193=DIRECTION ( 'NONE',  ( -1.550910762415566494E-16, -1.000000000000000000, 8.135128085091684243E-31 ) ) ;
#14196=VECTOR ( 'NONE', #7302, 1000.000000000000000 ) ;
#14210=CIRCLE ( 'NONE', #11938, 2.500000000000015987 ) ;
#14216=CARTESIAN_POINT ( 'NONE',  ( -55.05572809000119605, -1.179611963664228824E-13, -8.000000000000090594 ) ) ;
#14238=LINE ( 'NONE', #1310, #22208 ) ;
#14248=AXIS2_PLACEMENT_3D ( 'NONE', #19826, #3705, #5253 ) ;
#14249=CARTESIAN_POINT ( 'NONE',  ( -61.45000000000046469, 3.200000000000057465, -1.999999999999973577 ) ) ;
#14251=ORIENTED_EDGE ( 'NONE', *, *, #16953, .T. ) ;
#14253=ORIENTED_EDGE ( 'NONE', *, *, #17578, .T. ) ;
#14255=ORIENTED_EDGE ( 'NONE', *, *, #8659, .F. ) ;
#14259=DIRECTION ( 'NONE',  ( 1.000000000000000000, 0.000000000000000000, 0.000000000000000000 ) ) ;
#14260=EDGE_CURVE ( 'NONE', #11952, #16292, #18055, .T. ) ;
#14264=FACE_OUTER_BOUND ( 'NONE', #12535, .T. ) ;
#14271=CARTESIAN_POINT ( 'NONE',  ( -6.000000000000116351, 4.799999999999957190, -7.500000000000062172 ) ) ;
#14273=DIRECTION ( 'NONE',  ( 0.000000000000000000, 0.000000000000000000, -1.000000000000000000 ) ) ;
#14277=CARTESIAN_POINT ( 'NONE',  ( -6.000000000000116351, 1.999999999999960032, -7.500000000000062172 ) ) ;
#14280=EDGE_LOOP ( 'NONE', ( #6125, #12231, #4868, #22405 ) ) ;
#14286=CIRCLE ( 'NONE', #22159, 2.550000000000010481 ) ;
#14288=EDGE_CURVE ( 'NONE', #16175, #21212, #18801, .T. ) ;
#14297=DIRECTION ( 'NONE',  ( -2.013525853228508439E-32, -6.779273404243028164E-31, 1.000000000000000000 ) ) ;
#14304=DIRECTION ( 'NONE',  ( 0.000000000000000000, 0.000000000000000000, -1.000000000000000000 ) ) ;
#14308=CARTESIAN_POINT ( 'NONE',  ( -3.199999999999953104, -1.999999999999980904, -8.000000000000035527 ) ) ;
#14309=CARTESIAN_POINT ( 'NONE',  ( -89.70000000000064233, 2.700000000000056577, -2.000000000000001776 ) ) ;
#14312=ORIENTED_EDGE ( 'NONE', *, *, #16659, .T. ) ;
#14318=DIRECTION ( 'NONE',  ( -0.7071067811865536790, 0.7071067811865413555, 0.000000000000000000 ) ) ;
#14319=DIRECTION ( 'NONE',  ( -1.000000000000000000, -1.424116703980846297E-16, 1.095779650622964657E-32 ) ) ;
#14331=CIRCLE ( 'NONE', #15050, 0.4999999999999997224 ) ;
#14334=CARTESIAN_POINT ( 'NONE',  ( -57.28378781035996070, 9.020562075079396891E-14, 8.541666666666724694 ) ) ;
#14335=VERTEX_POINT ( 'NONE', #8126 ) ;
#14338=DIRECTION ( 'NONE',  ( 2.013525853228507892E-32, 6.902532920683810383E-31, -1.000000000000000000 ) ) ;
#14341=DIRECTION ( 'NONE',  ( -1.000000000000000000, 1.550910762415566494E-16, 6.133276141584333908E-48 ) ) ;
#14342=CIRCLE ( 'NONE', #12074, 9.500000000000056843 ) ;
#14343=VECTOR ( 'NONE', #936, 1000.000000000000000 ) ;
#14349=DIRECTION ( 'NONE',  ( 2.013525853228507892E-32, 6.902532920683810383E-31, -1.000000000000000000 ) ) ;
#14353=EDGE_CURVE ( 'NONE', #16829, #4291, #20719, .T. ) ;
#14355=ORIENTED_EDGE ( 'NONE', *, *, #8889, .F. ) ;
#14360=VECTOR ( 'NONE', #3951, 1000.000000000000000 ) ;
#14366=CYLINDRICAL_SURFACE ( 'NONE', #10265, 2.550000000000010481 ) ;
#14367=DIRECTION ( 'NONE',  ( 0.000000000000000000, 4.336808689941991704E-15, 1.000000000000000000 ) ) ;
#14373=CARTESIAN_POINT ( 'NONE',  ( -50.65685424949281668, 2.700000000000021938, 7.500000000000034639 ) ) ;
#14375=CARTESIAN_POINT ( 'NONE',  ( -65.00000000000044054, -3.200000000000088107, 2.999999999999947153 ) ) ;
#14381=AXIS2_PLACEMENT_3D ( 'NONE', #6914, #17607, #21033 ) ;
#14382=DIRECTION ( 'NONE',  ( -1.000000000000000000, 1.550910762415469612E-16, 0.000000000000000000 ) ) ;
#14392=EDGE_CURVE ( 'NONE', #18197, #7574, #16916, .T. ) ;
#14396=EDGE_LOOP ( 'NONE', ( #8869, #14905, #5545, #22092 ) ) ;
#14398=AXIS2_PLACEMENT_3D ( 'NONE', #12725, #23105, #17799 ) ;
#14401=CIRCLE ( 'NONE', #137, 0.4999999999999994449 ) ;
#14402=VERTEX_POINT ( 'NONE', #837 ) ;
#14406=CARTESIAN_POINT ( 'NONE',  ( -95.70000000000069917, 2.700000000000014833, -2.000000000000001776 ) ) ;
#14409=DIRECTION ( 'NONE',  ( 2.013525853228507892E-32, 6.902532920683810383E-31, -1.000000000000000000 ) ) ;
#14410=DIRECTION ( 'NONE',  ( -1.000000000000000000, 1.550910762415566494E-16, -2.686847401719668638E-48 ) ) ;
#14420=CIRCLE ( 'NONE', #4255, 0.5000000000000029976 ) ;
#14423=ORIENTED_EDGE ( 'NONE', *, *, #23086, .F. ) ;
#14426=ADVANCED_FACE ( 'NONE', ( #2703 ), #6132, .T. ) ;
#14442=CARTESIAN_POINT ( 'NONE',  ( -55.05572809000125289, 1.387778780781445676E-14, -10.00000000000006395 ) ) ;
#14457=VERTEX_POINT ( 'NONE', #8591 ) ;
#14459=ORIENTED_EDGE ( 'NONE', *, *, #9991, .T. ) ;
#14468=ORIENTED_EDGE ( 'NONE', *, *, #1904, .F. ) ;
#14469=DIRECTION ( 'NONE',  ( -1.000000000000000000, -2.220446049250314067E-16, 5.825996348268307008E-33 ) ) ;
#14473=DIRECTION ( 'NONE',  ( -1.000000000000000000, 2.168404344970992105E-16, -8.673617379883968419E-16 ) ) ;
#14474=PLANE ( 'NONE',  #1785 ) ;
#14477=DIRECTION ( 'NONE',  ( 2.220446049250313081E-16, -1.000000000000000000, 7.025792437124636392E-31 ) ) ;
#14478=DIRECTION ( 'NONE',  ( -1.000000000000000000, -2.220446049250314067E-16, 5.825996348268307008E-33 ) ) ;
#14483=ORIENTED_EDGE ( 'NONE', *, *, #13179, .T. ) ;
#14488=DIRECTION ( 'NONE',  ( -1.000000000000000000, -2.220446049250301001E-16, 0.000000000000000000 ) ) ;
#14496=DIRECTION ( 'NONE',  ( -2.013525853228507892E-32, -6.902532920683810383E-31, 1.000000000000000000 ) ) ;
#14503=ORIENTED_EDGE ( 'NONE', *, *, #1339, .T. ) ;
#14509=ORIENTED_EDGE ( 'NONE', *, *, #12592, .T. ) ;
#14513=ORIENTED_EDGE ( 'NONE', *, *, #18875, .F. ) ;
#14518=VECTOR ( 'NONE', #17238, 1000.000000000000000 ) ;
#14520=DIRECTION ( 'NONE',  ( -0.9706398123736329486, -2.155253336630096955E-16, -0.2405376366294442458 ) ) ;
#14531=ORIENTED_EDGE ( 'NONE', *, *, #1979, .F. ) ;
#14533=AXIS2_PLACEMENT_3D ( 'NONE', #20269, #14618, #10958 ) ;
#14536=ORIENTED_EDGE ( 'NONE', *, *, #11696, .F. ) ;
#14540=CARTESIAN_POINT ( 'NONE',  ( -45.56568542494948559, -2.108831175456959972, 7.500000000000076383 ) ) ;
#14546=DIRECTION ( 'NONE',  ( -1.000000000000000000, 1.550910762415526064E-16, 0.000000000000000000 ) ) ;
#14552=DIRECTION ( 'NONE',  ( 2.220446049250313081E-16, -1.000000000000000000, 7.025792437124636392E-31 ) ) ;
#14555=EDGE_CURVE ( 'NONE', #1883, #21928, #14238, .T. ) ;
#14560=ORIENTED_EDGE ( 'NONE', *, *, #17416, .T. ) ;
#14561=CIRCLE ( 'NONE', #7079, 3.300000000000020250 ) ;
#14563=CARTESIAN_POINT ( 'NONE',  ( -50.65685424949267457, -3.200000000000108979, -7.500000000000034639 ) ) ;
#14564=DIRECTION ( 'NONE',  ( -0.7071067811865580088, -0.7071067811865372477, 0.000000000000000000 ) ) ;
#14572=CARTESIAN_POINT ( 'NONE',  ( -50.65685424949274562, -7.200000000000077449, 8.000000000000062172 ) ) ;
#14575=ADVANCED_FACE ( 'NONE', ( #21541 ), #11043, .F. ) ;
#14580=DIRECTION ( 'NONE',  ( -4.336808689942045346E-15, 1.000000000000000000, 7.518830502887770522E-31 ) ) ;
#14583=PLANE ( 'NONE',  #17171 ) ;
#14590=CYLINDRICAL_SURFACE ( 'NONE', #16074, 2.550000000000010481 ) ;
#14592=EDGE_CURVE ( 'NONE', #5384, #477, #5424, .T. ) ;
#14593=AXIS2_PLACEMENT_3D ( 'NONE', #16656, #14903, #22089 ) ;
#14599=ORIENTED_EDGE ( 'NONE', *, *, #19999, .F. ) ;
#14602=CARTESIAN_POINT ( 'NONE',  ( -89.70000000000055707, -2.700000000000084110, -1.999999999999946265 ) ) ;
#14605=DIRECTION ( 'NONE',  ( 0.000000000000000000, 1.000000000000000000, 0.000000000000000000 ) ) ;
#14608=CIRCLE ( 'NONE', #21756, 2.550000000000010481 ) ;
#14617=DIRECTION ( 'NONE',  ( -0.7071067811865441310, -0.7071067811865510144, 0.000000000000000000 ) ) ;
#14618=DIRECTION ( 'NONE',  ( 1.550910762415566494E-16, 1.000000000000000000, -8.135128085091684243E-31 ) ) ;
#14623=EDGE_LOOP ( 'NONE', ( #10027, #9822, #3433, #19784 ) ) ;
#14627=ORIENTED_EDGE ( 'NONE', *, *, #17713, .T. ) ;
#14629=EDGE_LOOP ( 'NONE', ( #8987, #8871, #10518, #4456 ) ) ;
#14640=DIRECTION ( 'NONE',  ( 0.7071067811865535679, 0.7071067811865414665, 0.000000000000000000 ) ) ;
#14644=CARTESIAN_POINT ( 'NONE',  ( -56.91911807125113398, 0.5000000000000143219, -8.333333333333387216 ) ) ;
#14665=CARTESIAN_POINT ( 'NONE',  ( -50.65685424949274562, 2.700000000000021938, -8.000000000000062172 ) ) ;
#14666=FACE_OUTER_BOUND ( 'NONE', #1524, .T. ) ;
#14676=LINE ( 'NONE', #9501, #1962 ) ;
#14678=ORIENTED_EDGE ( 'NONE', *, *, #22824, .F. ) ;
#14679=CARTESIAN_POINT ( 'NONE',  ( -6.000000000000088818, 1.999999999999960032, -17.72029585817558228 ) ) ;
#14684=DIRECTION ( 'NONE',  ( -1.000000000000000000, 0.000000000000000000, 0.000000000000000000 ) ) ;
#14692=CARTESIAN_POINT ( 'NONE',  ( -43.06238456605044007, 5.319238815542546739, -8.000000000000090594 ) ) ;
#14695=EDGE_CURVE ( 'NONE', #8098, #18939, #19645, .T. ) ;
#14700=ORIENTED_EDGE ( 'NONE', *, *, #2092, .F. ) ;
#14715=PLANE ( 'NONE',  #16632 ) ;
#14721=CARTESIAN_POINT ( 'NONE',  ( -6.000000000000143885, 1.999999999999960032, 8.000000000000062172 ) ) ;
#14723=VECTOR ( 'NONE', #10949, 1000.000000000000000 ) ;
#14730=EDGE_LOOP ( 'NONE', ( #33, #13501, #2411, #12982 ) ) ;
#14738=ADVANCED_FACE ( 'NONE', ( #22345 ), #22222, .T. ) ;
#14748=LINE ( 'NONE', #16613, #18506 ) ;
#14762=AXIS2_PLACEMENT_3D ( 'NONE', #990, #15661, #6511 ) ;
#14765=ORIENTED_EDGE ( 'NONE', *, *, #12022, .F. ) ;
#14767=VECTOR ( 'NONE', #14520, 1000.000000000000114 ) ;
#14770=EDGE_LOOP ( 'NONE', ( #14018, #22822, #5380, #12569 ) ) ;
#14776=CARTESIAN_POINT ( 'NONE',  ( -6.000000000000116351, 7.499999999999958256, -7.500000000000062172 ) ) ;
#14785=CIRCLE ( 'NONE', #158, 0.5000000000000029976 ) ;
#14786=AXIS2_PLACEMENT_3D ( 'NONE', #16121, #12477, #377 ) ;
#14788=CARTESIAN_POINT ( 'NONE',  ( -47.82842712474642610, -4.371572875253856516, 8.000000000000076383 ) ) ;
#14798=FACE_OUTER_BOUND ( 'NONE', #21723, .T. ) ;
#14809=DIRECTION ( 'NONE',  ( -2.220446049250313081E-16, 1.000000000000000000, -7.025792437124636392E-31 ) ) ;
#14824=VERTEX_POINT ( 'NONE', #1054 ) ;
#14828=ORIENTED_EDGE ( 'NONE', *, *, #1810, .T. ) ;
#14844=ADVANCED_FACE ( 'NONE', ( #7749 ), #5878, .F. ) ;
#14846=VECTOR ( 'NONE', #10326, 1000.000000000000000 ) ;
#14850=ORIENTED_EDGE ( 'NONE', *, *, #11456, .T. ) ;
#14854=ORIENTED_EDGE ( 'NONE', *, *, #474, .T. ) ;
#14860=ORIENTED_EDGE ( 'NONE', *, *, #20127, .F. ) ;
#14865=ADVANCED_FACE ( 'NONE', ( #20696 ), #19585, .T. ) ;
#14867=EDGE_CURVE ( 'NONE', #7024, #7626, #5691, .T. ) ;
#14869=EDGE_CURVE ( 'NONE', #6492, #6466, #9444, .T. ) ;
#14873=FILL_AREA_STYLE_COLOUR ( '', #15094 ) ;
#14879=ORIENTED_EDGE ( 'NONE', *, *, #14002, .T. ) ;
#14887=EDGE_LOOP ( 'NONE', ( #4225, #10776, #16658, #16394, #1884, #4027, #2441, #1239, #6011, #18300, #3765, #3736 ) ) ;
#14888=DIRECTION ( 'NONE',  ( 1.000000000000000000, 0.000000000000000000, 0.000000000000000000 ) ) ;
#14890=VERTEX_POINT ( 'NONE', #13964 ) ;
#14894=CARTESIAN_POINT ( 'NONE',  ( -91.02295700146262902, 0.5000000000000073275, 6.338518968055040226 ) ) ;
#14896=LINE ( 'NONE', #14665, #4915 ) ;
#14897=FACE_OUTER_BOUND ( 'NONE', #9793, .T. ) ;
#14899=DIRECTION ( 'NONE',  ( 2.013525853228507892E-32, 6.902532920683810383E-31, -1.000000000000000000 ) ) ;
#14900=EDGE_CURVE ( 'NONE', #6614, #3480, #18458, .T. ) ;
#14903=DIRECTION ( 'NONE',  ( 1.298062744027682297E-32, -6.902532920683810383E-31, 1.000000000000000000 ) ) ;
#14905=ORIENTED_EDGE ( 'NONE', *, *, #19882, .F. ) ;
#14907=EDGE_LOOP ( 'NONE', ( #19055, #21591, #14850, #19051 ) ) ;
#14908=DIRECTION ( 'NONE',  ( -0.1556420233463033653, 0.000000000000000000, -0.9878135252003128475 ) ) ;
#14919=DIRECTION ( 'NONE',  ( -2.220446049250313081E-16, 1.000000000000000000, -7.025792437124636392E-31 ) ) ;
#14920=AXIS2_PLACEMENT_3D ( 'NONE', #20363, #20258, #2251 ) ;
#14921=DIRECTION ( 'NONE',  ( 1.000000000000000000, 1.424116703980846297E-16, -1.095779650622964657E-32 ) ) ;
#14933=VERTEX_POINT ( 'NONE', #23041 ) ;
#14962=AXIS2_PLACEMENT_3D ( 'NONE', #15185, #16824, #4720 ) ;
#14968=EDGE_LOOP ( 'NONE', ( #2969, #311, #17684, #13499 ) ) ;
#14972=EDGE_LOOP ( 'NONE', ( #6151, #21364, #1205, #16060 ) ) ;
#14984=SURFACE_SIDE_STYLE ('',( #9586 ) ) ;
#14993=EDGE_CURVE ( 'NONE', #15165, #7024, #7563, .T. ) ;
#15001=EDGE_CURVE ( 'NONE', #16292, #16331, #13200, .T. ) ;
#15005=CARTESIAN_POINT ( 'NONE',  ( -1.110223024625156540E-13, 1.999999999999932498, 7.500000000000034639 ) ) ;
#15006=DIRECTION ( 'NONE',  ( 1.000000000000000000, 2.220446049250313081E-16, 4.712618736834399899E-47 ) ) ;
#15010=DIRECTION ( 'NONE',  ( 2.013525853228507892E-32, 6.902532920683810383E-31, -1.000000000000000000 ) ) ;
#15011=AXIS2_PLACEMENT_3D ( 'NONE', #5245, #21006, #21124 ) ;
#15013=PLANE ( 'NONE',  #1738 ) ;
#15019=VERTEX_POINT ( 'NONE', #18087 ) ;
#15021=DIRECTION ( 'NONE',  ( -0.7071067811865412445, 0.7071067811865539010, 1.565905175853772837E-16 ) ) ;
#15023=AXIS2_PLACEMENT_3D ( 'NONE', #155, #7327, #10943 ) ;
#15026=LINE ( 'NONE', #7517, #5508 ) ;
#15034=CARTESIAN_POINT ( 'NONE',  ( -64.00000000000045475, -7.632783294297951215E-14, -2.000000000000001776 ) ) ;
#15045=ADVANCED_BREP_SHAPE_REPRESENTATION ( '', ( #5304, #22115 ), #12708 ) ;
#15049=AXIS2_PLACEMENT_3D ( 'NONE', #3647, #5651, #21430 ) ;
#15050=AXIS2_PLACEMENT_3D ( 'NONE', #13723, #17703, #23011 ) ;
#15056=CARTESIAN_POINT ( 'NONE',  ( -45.56568542494957086, 2.108831175456883589, 7.500000000000047962 ) ) ;
#15061=LINE ( 'NONE', #506, #12300 ) ;
#15063=DIRECTION ( 'NONE',  ( -0.7453559924999295649, 0.000000000000000000, 0.6666666666666669627 ) ) ;
#15064=ORIENTED_EDGE ( 'NONE', *, *, #21051, .F. ) ;
#15067=ORIENTED_EDGE ( 'NONE', *, *, #13004, .T. ) ;
#15069=EDGE_LOOP ( 'NONE', ( #12177, #17815, #11786, #22335 ) ) ;
#15074=DIRECTION ( 'NONE',  ( -0.7071067811865539010, -0.7071067811865413555, 0.000000000000000000 ) ) ;
#15085=AXIS2_PLACEMENT_3D ( 'NONE', #13163, #7158, #14318 ) ;
#15089=DIRECTION ( 'NONE',  ( -1.000000000000000000, 0.000000000000000000, 0.000000000000000000 ) ) ;
#15092=VERTEX_POINT ( 'NONE', #15229 ) ;
#15094=COLOUR_RGB ( '', 0.40784314, 0.44705882, 0.49803922) ;
#15098=ORIENTED_EDGE ( 'NONE', *, *, #13532, .T. ) ;
#15099=EDGE_CURVE ( 'NONE', #4862, #12385, #2686, .T. ) ;
#15100=ORIENTED_EDGE ( 'NONE', *, *, #5701, .F. ) ;
#15101=CIRCLE ( 'NONE', #13987, 5.500000000000033751 ) ;
#15103=ORIENTED_EDGE ( 'NONE', *, *, #3528, .F. ) ;
#15108=ORIENTED_EDGE ( 'NONE', *, *, #15978, .F. ) ;
#15122=CARTESIAN_POINT ( 'NONE',  ( -43.10883117545713361, -4.565685424949276872, 8.000000000000035527 ) ) ;
#15136=ORIENTED_EDGE ( 'NONE', *, *, #11228, .F. ) ;
#15137=ADVANCED_FACE ( 'NONE', ( #6076 ), #16880, .T. ) ;
#15148=CARTESIAN_POINT ( 'NONE',  ( -42.54314575050796776, 4.799999999999991829, -8.000000000000035527 ) ) ;
#15149=VECTOR ( 'NONE', #8610, 1000.000000000000000 ) ;
#15165=VERTEX_POINT ( 'NONE', #2657 ) ;
#15173=AXIS2_PLACEMENT_3D ( 'NONE', #15560, #12020, #17083 ) ;
#15185=CARTESIAN_POINT ( 'NONE',  ( -50.65685424949280247, -0.5000000000001045830, 7.500000000000062172 ) ) ;
#15188=ORIENTED_EDGE ( 'NONE', *, *, #21882, .T. ) ;
#15189=VECTOR ( 'NONE', #22720, 1000.000000000000000 ) ;
#15195=ORIENTED_EDGE ( 'NONE', *, *, #20885, .F. ) ;
#15196=VERTEX_POINT ( 'NONE', #5857 ) ;
#15197=ORIENTED_EDGE ( 'NONE', *, *, #14592, .T. ) ;
#15198=CARTESIAN_POINT ( 'NONE',  ( -42.54314575050778302, -7.500000000000020428, 7.500000000000034639 ) ) ;
#15213=EDGE_LOOP ( 'NONE', ( #14251, #7200, #22091, #16299 ) ) ;
#15219=ORIENTED_EDGE ( 'NONE', *, *, #11027, .T. ) ;
#15224=EDGE_LOOP ( 'NONE', ( #16262, #4554, #22733, #7797 ) ) ;
#15229=CARTESIAN_POINT ( 'NONE',  ( -43.10883117545713361, -4.565685424949256443, -7.500000000000007105 ) ) ;
#15232=FACE_OUTER_BOUND ( 'NONE', #9137, .T. ) ;
#15237=AXIS2_PLACEMENT_3D ( 'NONE', #21791, #16234, #21332 ) ;
#15242=ADVANCED_FACE ( 'NONE', ( #6654 ), #6827, .T. ) ;
#15244=VERTEX_POINT ( 'NONE', #22545 ) ;
#15248=DIRECTION ( 'NONE',  ( 0.1556420233463076119, 0.000000000000000000, 0.9878135252003121813 ) ) ;
#15262=LINE ( 'NONE', #13286, #11075 ) ;
#15269=ADVANCED_FACE ( 'NONE', ( #19233 ), #19973, .T. ) ;
#15273=ORIENTED_EDGE ( 'NONE', *, *, #11667, .T. ) ;
#15274=EDGE_CURVE ( 'NONE', #11922, #8762, #14342, .T. ) ;
#15279=CIRCLE ( 'NONE', #15664, 0.5000000000000029976 ) ;
#15288=EDGE_CURVE ( 'NONE', #10662, #16835, #10580, .T. ) ;
#15292=DIRECTION ( 'NONE',  ( -1.000000000000000000, 1.550910762415508562E-16, 0.000000000000000000 ) ) ;
#15295=CARTESIAN_POINT ( 'NONE',  ( -6.000000000000074607, 5.299999999999964295, 7.500000000000062172 ) ) ;
#15300=FACE_OUTER_BOUND ( 'NONE', #7715, .T. ) ;
#15301=CARTESIAN_POINT ( 'NONE',  ( -50.65685424949273141, 0.5000000000000143219, 8.000000000000076383 ) ) ;
#15309=EDGE_LOOP ( 'NONE', ( #22028, #17721, #10936, #22969 ) ) ;
#15324=AXIS2_PLACEMENT_3D ( 'NONE', #11867, #13868, #19270 ) ;
#15325=CYLINDRICAL_SURFACE ( 'NONE', #11429, 0.5000000000000037748 ) ;
#15333=DIRECTION ( 'NONE',  ( 0.7071067811865505703, -0.7071067811865444641, -1.010793663541190129E-16 ) ) ;
#15344=AXIS2_PLACEMENT_3D ( 'NONE', #5711, #7582, #292 ) ;
#15351=CARTESIAN_POINT ( 'NONE',  ( -89.70000000000048601, -3.200000000000105427, 1.000000000000000888 ) ) ;
#15352=DIRECTION ( 'NONE',  ( 1.000000000000000000, 1.424116703980846297E-16, -1.095779650622964657E-32 ) ) ;
#15354=VECTOR ( 'NONE', #1415, 1000.000000000000000 ) ;
#15355=DIRECTION ( 'NONE',  ( 1.000000000000000000, 2.220446049250313081E-16, -3.656342123407315983E-48 ) ) ;
#15358=CARTESIAN_POINT ( 'NONE',  ( -56.54644007500113645, 1.387778780781445676E-14, -8.666666666666710483 ) ) ;
#15359=TOROIDAL_SURFACE ( 'NONE', #9749, 5.500000000000007994, 0.5000000000000000000 ) ;
#15361=LINE ( 'NONE', #22551, #14518 ) ;
#15377=CARTESIAN_POINT ( 'NONE',  ( -6.866595637048056311, 0.5000000000001045830, 27.70872448147268585 ) ) ;
#15383=CARTESIAN_POINT ( 'NONE',  ( -91.02295700146254376, -2.700000000000125855, 6.338518968055040226 ) ) ;
#15401=CARTESIAN_POINT ( 'NONE',  ( -43.10883117545721888, 4.565685424949256443, -7.500000000000034639 ) ) ;
#15404=DIRECTION ( 'NONE',  ( -1.000000000000000000, -1.479114197289388027E-30, 2.013525853228518840E-32 ) ) ;
#15409=CARTESIAN_POINT ( 'NONE',  ( -50.65685424949273141, 7.200000000000025935, 8.000000000000076383 ) ) ;
#15411=DIRECTION ( 'NONE',  ( -1.000000000000000000, 1.550910762415566494E-16, -8.566929763922626680E-48 ) ) ;
#15412=LINE ( 'NONE', #22840, #7091 ) ;
#15418=LINE ( 'NONE', #8259, #7404 ) ;
#15423=EDGE_CURVE ( 'NONE', #10146, #16829, #1589, .T. ) ;
#15431=ADVANCED_FACE ( 'NONE', ( #12282 ), #5121, .T. ) ;
#15444=AXIS2_PLACEMENT_3D ( 'NONE', #6454, #3165, #17617 ) ;
#15446=CARTESIAN_POINT ( 'NONE',  ( -45.91923881554281195, -2.462384566050190848, -8.000000000000062172 ) ) ;
#15459=CIRCLE ( 'NONE', #1204, 0.5000000000000024425 ) ;
#15466=CARTESIAN_POINT ( 'NONE',  ( -55.25320565519150051, 3.200000000000098765, 7.500000000000062172 ) ) ;
#15474=DIRECTION ( 'NONE',  ( -2.220446049250313081E-16, 1.000000000000000000, -7.025792437124636392E-31 ) ) ;
#15475=EDGE_LOOP ( 'NONE', ( #3365, #21081, #12807, #19162 ) ) ;
#15478=AXIS2_PLACEMENT_3D ( 'NONE', #14776, #787, #9833 ) ;
#15479=ORIENTED_EDGE ( 'NONE', *, *, #6379, .F. ) ;
#15483=ORIENTED_EDGE ( 'NONE', *, *, #2207, .F. ) ;
#15487=DIRECTION ( 'NONE',  ( -0.9878135252003119593, 5.399917434947377318E-16, 0.1556420233463085001 ) ) ;
#15489=VERTEX_POINT ( 'NONE', #15056 ) ;
#15494=AXIS2_PLACEMENT_3D ( 'NONE', #15351, #21125, #11703 ) ;
#15507=VECTOR ( 'NONE', #5479, 1000.000000000000000 ) ;
#15508=CIRCLE ( 'NONE', #16679, 0.5000000000000001110 ) ;
#15512=CIRCLE ( 'NONE', #18169, 0.8000000000000090372 ) ;
#15516=CARTESIAN_POINT ( 'NONE',  ( -65.47859922179033276, 4.857225732735059864E-14, -11.38422848940298593 ) ) ;
#15517=CYLINDRICAL_SURFACE ( 'NONE', #10339, 0.5000000000000004441 ) ;
#15535=EDGE_CURVE ( 'NONE', #18914, #2832, #8718, .T. ) ;
#15537=CARTESIAN_POINT ( 'NONE',  ( -42.54314575050793934, -4.800000000000019362, 7.500000000000062172 ) ) ;
#15541=ORIENTED_EDGE ( 'NONE', *, *, #11402, .F. ) ;
#15549=AXIS2_PLACEMENT_3D ( 'NONE', #19815, #12751, #9457 ) ;
#15554=CYLINDRICAL_SURFACE ( 'NONE', #22192, 6.000000000000047073 ) ;
#15558=CYLINDRICAL_SURFACE ( 'NONE', #7647, 2.550000000000010481 ) ;
#15559=CARTESIAN_POINT ( 'NONE',  ( -52.60445557845689990, 2.700000000000056577, 15.85914177512520773 ) ) ;
#15560=CARTESIAN_POINT ( 'NONE',  ( -6.000000000000088818, -8.000000000000042633, 8.000000000000062172 ) ) ;
#15570=EDGE_CURVE ( 'NONE', #19569, #21118, #22607, .T. ) ;
#15571=ORIENTED_EDGE ( 'NONE', *, *, #1818, .T. ) ;
#15576=VERTEX_POINT ( 'NONE', #20724 ) ;
#15584=CARTESIAN_POINT ( 'NONE',  ( -61.45000000000044338, -7.672331518739547608E-14, -2.000000000000002220 ) ) ;
#15585=CARTESIAN_POINT ( 'NONE',  ( -95.70000000000062812, -0.5000000000000975886, 8.000000000000062172 ) ) ;
#15587=CARTESIAN_POINT ( 'NONE',  ( -6.000000000000074607, 1.999999999999960032, 7.500000000000062172 ) ) ;
#15590=CARTESIAN_POINT ( 'NONE',  ( -50.65685424949273141, 7.200000000000025935, 8.000000000000076383 ) ) ;
#15608=AXIS2_PLACEMENT_3D ( 'NONE', #11132, #9261, #14546 ) ;
#15615=EDGE_CURVE ( 'NONE', #22415, #16051, #10581, .T. ) ;
#15621=DIRECTION ( 'NONE',  ( -2.220446049250313081E-16, 1.000000000000000000, -7.025792437124636392E-31 ) ) ;
#15638=DIRECTION ( 'NONE',  ( -0.7071067811865485719, 0.7071067811865464625, 1.010793663541191485E-16 ) ) ;
#15640=FACE_OUTER_BOUND ( 'NONE', #14043, .T. ) ;
#15641=FACE_OUTER_BOUND ( 'NONE', #17041, .T. ) ;
#15647=ORIENTED_EDGE ( 'NONE', *, *, #15709, .T. ) ;
#15654=EDGE_LOOP ( 'NONE', ( #6697, #14423, #6673, #10087 ) ) ;
#15661=DIRECTION ( 'NONE',  ( -2.013525853228507892E-32, -6.902532920683810383E-31, 1.000000000000000000 ) ) ;
#15664=AXIS2_PLACEMENT_3D ( 'NONE', #3545, #1661, #1874 ) ;
#15668=PLANE ( 'NONE',  #4383 ) ;
#15670=DIRECTION ( 'NONE',  ( 2.220446049250313081E-16, -1.000000000000000000, 7.025792437124636392E-31 ) ) ;
#15680=ADVANCED_FACE ( 'NONE', ( #21757 ), #4089, .T. ) ;
#15682=VERTEX_POINT ( 'NONE', #18333 ) ;
#15685=ORIENTED_EDGE ( 'NONE', *, *, #9053, .T. ) ;
#15707=ADVANCED_FACE ( 'NONE', ( #1971 ), #18096, .T. ) ;
#15708=AXIS2_PLACEMENT_3D ( 'NONE', #1766, #19890, #3758 ) ;
#15709=EDGE_CURVE ( 'NONE', #11317, #20537, #12478, .T. ) ;
#15714=ORIENTED_EDGE ( 'NONE', *, *, #4422, .F. ) ;
#15724=DIRECTION ( 'NONE',  ( -2.013525853228507892E-32, -6.902532920683810383E-31, 1.000000000000000000 ) ) ;
#15748=VECTOR ( 'NONE', #2949, 1000.000000000000000 ) ;
#15752=EDGE_CURVE ( 'NONE', #15826, #22801, #91, .T. ) ;
#15755=EDGE_LOOP ( 'NONE', ( #15790, #6103, #16725, #5912 ) ) ;
#15756=DIRECTION ( 'NONE',  ( -2.220446049250313081E-16, 1.000000000000000000, -7.025792437124636392E-31 ) ) ;
#15763=DIRECTION ( 'NONE',  ( 1.000000000000000000, 2.220446049250314067E-16, -5.825996348268307008E-33 ) ) ;
#15764=AXIS2_PLACEMENT_3D ( 'NONE', #20398, #6399, #7922 ) ;
#15779=DIRECTION ( 'NONE',  ( -1.000000000000000000, -1.700709290173333260E-16, 0.000000000000000000 ) ) ;
#15785=EDGE_CURVE ( 'NONE', #3212, #477, #3439, .T. ) ;
#15786=CARTESIAN_POINT ( 'NONE',  ( -50.65685424949274562, -1.040834085586084257E-13, 8.000000000000062172 ) ) ;
#15789=CARTESIAN_POINT ( 'NONE',  ( -50.65685424949280247, -1.040834085586084257E-13, 7.500000000000062172 ) ) ;
#15790=ORIENTED_EDGE ( 'NONE', *, *, #15901, .T. ) ;
#15791=VECTOR ( 'NONE', #126, 1000.000000000000000 ) ;
#15796=ORIENTED_EDGE ( 'NONE', *, *, #5106, .T. ) ;
#15801=ORIENTED_EDGE ( 'NONE', *, *, #16294, .F. ) ;
#15802=DIRECTION ( 'NONE',  ( -1.000000000000000000, 1.700709290173333260E-16, 0.000000000000000000 ) ) ;
#15807=CIRCLE ( 'NONE', #6070, 2.550000000000010481 ) ;
#15809=DIRECTION ( 'NONE',  ( 0.2405376366294550983, 0.000000000000000000, -0.9706398123736303951 ) ) ;
#15812=FACE_OUTER_BOUND ( 'NONE', #2878, .T. ) ;
#15821=EDGE_LOOP ( 'NONE', ( #11180, #9887, #19901, #3826 ) ) ;
#15826=VERTEX_POINT ( 'NONE', #2220 ) ;
#15835=CARTESIAN_POINT ( 'NONE',  ( -6.000000000000074607, 5.299999999999964295, 7.500000000000062172 ) ) ;
#15843=CARTESIAN_POINT ( 'NONE',  ( -55.25320565519145788, 2.700000000000098321, 10.00000000000009237 ) ) ;
#15847=ORIENTED_EDGE ( 'NONE', *, *, #4829, .T. ) ;
#15852=EDGE_LOOP ( 'NONE', ( #18525, #1401, #20301, #10062 ) ) ;
#15855=CARTESIAN_POINT ( 'NONE',  ( -43.10883117545713361, -4.565685424949276872, 8.000000000000035527 ) ) ;
#15866=DIRECTION ( 'NONE',  ( -1.550910762415566494E-16, -1.000000000000000000, 8.135128085091684243E-31 ) ) ;
#15869=EDGE_CURVE ( 'NONE', #19838, #21118, #12456, .T. ) ;
#15877=EDGE_CURVE ( 'NONE', #21725, #6466, #2318, .T. ) ;
#15878=ORIENTED_EDGE ( 'NONE', *, *, #10158, .F. ) ;
#15892=VECTOR ( 'NONE', #1792, 1000.000000000000000 ) ;
#15894=AXIS2_PLACEMENT_3D ( 'NONE', #20944, #1301, #8472 ) ;
#15896=EDGE_CURVE ( 'NONE', #7485, #3212, #15459, .T. ) ;
#15901=EDGE_CURVE ( 'NONE', #10886, #4366, #20693, .T. ) ;
#15902=DIRECTION ( 'NONE',  ( -2.013525853228507892E-32, -6.902532920683810383E-31, 1.000000000000000000 ) ) ;
#15906=ADVANCED_FACE ( 'NONE', ( #11381 ), #9510, .T. ) ;
#15921=CYLINDRICAL_SURFACE ( 'NONE', #1508, 7.200000000000046363 ) ;
#15927=AXIS2_PLACEMENT_3D ( 'NONE', #11995, #3071, #15411 ) ;
#15929=CARTESIAN_POINT ( 'NONE',  ( -3.200000000000119194, -6.938893903907228378E-14, 7.500000000000062172 ) ) ;
#15937=ORIENTED_EDGE ( 'NONE', *, *, #8834, .T. ) ;
#15940=VERTEX_POINT ( 'NONE', #6221 ) ;
#15943=AXIS2_PLACEMENT_3D ( 'NONE', #10585, #7187, #12343 ) ;
#15950=FACE_OUTER_BOUND ( 'NONE', #14396, .T. ) ;
#15960=CARTESIAN_POINT ( 'NONE',  ( -6.000000000000143885, -2.000000000000043521, 8.000000000000062172 ) ) ;
#15964=DIRECTION ( 'NONE',  ( -2.013525853228507892E-32, -6.902532920683810383E-31, 1.000000000000000000 ) ) ;
#15970=DIRECTION ( 'NONE',  ( 1.000000000000000000, -1.389842848855773151E-62, 2.013525853228507618E-32 ) ) ;
#15971=ORIENTED_EDGE ( 'NONE', *, *, #1959, .T. ) ;
#15972=ORIENTED_EDGE ( 'NONE', *, *, #8838, .F. ) ;
#15975=DIRECTION ( 'NONE',  ( 2.013525853228507892E-32, 6.902532920683810383E-31, -1.000000000000000000 ) ) ;
#15978=EDGE_CURVE ( 'NONE', #15576, #22415, #4947, .T. ) ;
#15979=ORIENTED_EDGE ( 'NONE', *, *, #3328, .T. ) ;
#15980=AXIS2_PLACEMENT_3D ( 'NONE', #5676, #3890, #3667 ) ;
#15984=DIRECTION ( 'NONE',  ( -2.220446049250313081E-16, 1.000000000000000000, -7.025792437124636392E-31 ) ) ;
#15989=DIRECTION ( 'NONE',  ( -0.2405376366294452728, 0.000000000000000000, 0.9706398123736327266 ) ) ;
#15998=AXIS2_PLACEMENT_3D ( 'NONE', #17756, #13992, #7178 ) ;
#16015=CARTESIAN_POINT ( 'NONE',  ( -55.25320565519145788, 0.5000000000000905942, 10.00000000000009237 ) ) ;
#16017=CARTESIAN_POINT ( 'NONE',  ( -95.70000000000058549, -2.700000000000119194, 1.000000000000014655 ) ) ;
#16021=DIRECTION ( 'NONE',  ( -1.000000000000000000, -2.220446049250301001E-16, 0.000000000000000000 ) ) ;
#16023=EDGE_CURVE ( 'NONE', #4862, #5668, #20926, .T. ) ;
#16028=VERTEX_POINT ( 'NONE', #10200 ) ;
#16031=ORIENTED_EDGE ( 'NONE', *, *, #67, .T. ) ;
#16035=DIRECTION ( 'NONE',  ( 0.9706398123736300620, 1.281898970984135951E-30, 0.2405376366294562085 ) ) ;
#16038=CARTESIAN_POINT ( 'NONE',  ( -3.414274948570356294, 6.938893903907228378E-14, -21.66938530120590656 ) ) ;
#16041=CARTESIAN_POINT ( 'NONE',  ( -89.70000000000055707, -2.700000000000084110, -1.999999999999946265 ) ) ;
#16048=CIRCLE ( 'NONE', #6679, 4.500000000000031974 ) ;
#16049=CARTESIAN_POINT ( 'NONE',  ( -65.47859922179024750, -3.200000000000088107, -11.38422848940306942 ) ) ;
#16051=VERTEX_POINT ( 'NONE', #6922 ) ;
#16057=CIRCLE ( 'NONE', #22087, 0.5000000000000029976 ) ;
#16060=ORIENTED_EDGE ( 'NONE', *, *, #8222, .F. ) ;
#16061=ORIENTED_EDGE ( 'NONE', *, *, #7959, .T. ) ;
#16066=CIRCLE ( 'NONE', #19085, 0.5000000000000006661 ) ;
#16074=AXIS2_PLACEMENT_3D ( 'NONE', #21662, #16218, #21315 ) ;
#16075=DIRECTION ( 'NONE',  ( 1.000000000000000000, 0.000000000000000000, 0.000000000000000000 ) ) ;
#16076=AXIS2_PLACEMENT_3D ( 'NONE', #21661, #5186, #19534 ) ;
#16086=CARTESIAN_POINT ( 'NONE',  ( -56.87767137932630845, 0.5000000000000905942, 8.833333333333415638 ) ) ;
#16087=AXIS2_PLACEMENT_3D ( 'NONE', #4184, #12914, #2083 ) ;
#16109=EDGE_CURVE ( 'NONE', #8762, #12385, #5145, .T. ) ;
#16117=ORIENTED_EDGE ( 'NONE', *, *, #6360, .F. ) ;
#16121=CARTESIAN_POINT ( 'NONE',  ( -67.28510754798017501, -0.5000000000001045830, 12.22107821754960000 ) ) ;
#16126=DIRECTION ( 'NONE',  ( 0.000000000000000000, 0.000000000000000000, 1.000000000000000000 ) ) ;
#16129=DIRECTION ( 'NONE',  ( -0.7071067811865233699, 0.7071067811865715536, 1.565905175853783930E-16 ) ) ;
#16150=EDGE_LOOP ( 'NONE', ( #22181, #571, #14860, #274 ) ) ;
#16154=CARTESIAN_POINT ( 'NONE',  ( -50.65685424949267457, -3.200000000000108979, -7.500000000000034639 ) ) ;
#16163=CARTESIAN_POINT ( 'NONE',  ( -57.28378781035996070, 3.200000000000098765, 8.541666666666724694 ) ) ;
#16169=CARTESIAN_POINT ( 'NONE',  ( -92.25000000000058265, -8.981013850637800498E-14, -2.000000000000001776 ) ) ;
#16175=VERTEX_POINT ( 'NONE', #14540 ) ;
#16176=ORIENTED_EDGE ( 'NONE', *, *, #779, .T. ) ;
#16177=DIRECTION ( 'NONE',  ( 0.9706398123736330597, 2.155253336630096709E-16, 0.2405376366294442736 ) ) ;
#16179=CARTESIAN_POINT ( 'NONE',  ( -0.5000000000000837108, 7.199999999999977085, -8.000000000000007105 ) ) ;
#16180=ADVANCED_FACE ( 'NONE', ( #12658 ), #7379, .T. ) ;
#16189=CARTESIAN_POINT ( 'NONE',  ( -6.866595637047972822, -0.5000000000000350830, 27.70872448147272848 ) ) ;
#16190=DIRECTION ( 'NONE',  ( -2.220446049250313081E-16, 1.000000000000000000, -7.025792437124636392E-31 ) ) ;
#16194=DIRECTION ( 'NONE',  ( -2.013525853228518840E-32, 6.902532920683810383E-31, -1.000000000000000000 ) ) ;
#16195=AXIS2_PLACEMENT_3D ( 'NONE', #19849, #10894, #9260 ) ;
#16200=ORIENTED_EDGE ( 'NONE', *, *, #12953, .F. ) ;
#16218=DIRECTION ( 'NONE',  ( -2.220446049250313081E-16, 1.000000000000000000, -7.025792437124636392E-31 ) ) ;
#16222=VERTEX_POINT ( 'NONE', #18084 ) ;
#16224=TOROIDAL_SURFACE ( 'NONE', #1226, 1.300000000000000711, 0.5000000000000000000 ) ;
#16234=DIRECTION ( 'NONE',  ( 2.013525853228518840E-32, -6.902532920683810383E-31, 1.000000000000000000 ) ) ;
#16238=DIRECTION ( 'NONE',  ( 1.000000000000000000, 0.000000000000000000, 0.000000000000000000 ) ) ;
#16239=ADVANCED_FACE ( 'NONE', ( #10670 ), #17853, .T. ) ;
#16246=VECTOR ( 'NONE', #16960, 1000.000000000000000 ) ;
#16251=ORIENTED_EDGE ( 'NONE', *, *, #12256, .T. ) ;
#16254=ORIENTED_EDGE ( 'NONE', *, *, #5082, .T. ) ;
#16258=CIRCLE ( 'NONE', #8014, 2.500000000000015987 ) ;
#16262=ORIENTED_EDGE ( 'NONE', *, *, #18294, .F. ) ;
#16266=ORIENTED_EDGE ( 'NONE', *, *, #22163, .F. ) ;
#16270=CARTESIAN_POINT ( 'NONE',  ( -6.000000000000074607, -5.300000000000023803, -7.500000000000034639 ) ) ;
#16274=EDGE_CURVE ( 'NONE', #20569, #21208, #18312, .T. ) ;
#16276=CARTESIAN_POINT ( 'NONE',  ( -55.25320565519142946, -0.5000000000000281997, 8.000000000000076383 ) ) ;
#16282=FACE_OUTER_BOUND ( 'NONE', #15069, .T. ) ;
#16284=DIRECTION ( 'NONE',  ( -1.000000000000000000, 1.389842848855773367E-62, -2.013525853228507892E-32 ) ) ;
#16285=VECTOR ( 'NONE', #21151, 1000.000000000000000 ) ;
#16292=VERTEX_POINT ( 'NONE', #20427 ) ;
#16294=EDGE_CURVE ( 'NONE', #22801, #9172, #2422, .T. ) ;
#16296=ADVANCED_FACE ( 'NONE', ( #11245 ), #668, .T. ) ;
#16299=ORIENTED_EDGE ( 'NONE', *, *, #6870, .T. ) ;
#16300=CARTESIAN_POINT ( 'NONE',  ( -42.54314575050785407, -4.000000000000034639, -7.500000000000007105 ) ) ;
#16309=DIRECTION ( 'NONE',  ( 2.220446049250313081E-16, -1.000000000000000000, 7.025792437124636392E-31 ) ) ;
#16320=PLANE ( 'NONE',  #8545 ) ;
#16323=FACE_OUTER_BOUND ( 'NONE', #16470, .T. ) ;
#16331=VERTEX_POINT ( 'NONE', #22420 ) ;
#16336=EDGE_CURVE ( 'NONE', #22532, #7024, #13018, .T. ) ;
#16364=PLANE ( 'NONE',  #2513 ) ;
#16372=ORIENTED_EDGE ( 'NONE', *, *, #761, .T. ) ;
#16374=UNCERTAINTY_MEASURE_WITH_UNIT (LENGTH_MEASURE( 1.000000000000000082E-05 ), #6176, 'distance_accuracy_value', 'NONE');
#16378=ORIENTED_EDGE ( 'NONE', *, *, #19165, .F. ) ;
#16383=DIRECTION ( 'NONE',  ( -1.000000000000000000, -1.479114197289388027E-30, 2.013525853228518840E-32 ) ) ;
#16384=CARTESIAN_POINT ( 'NONE',  ( -87.15000000000063096, 5.607736497381665307E-14, -2.000000000000001332 ) ) ;
#16390=DIRECTION ( 'NONE',  ( -0.7453559924999295649, 0.000000000000000000, 0.6666666666666669627 ) ) ;
#16392=CARTESIAN_POINT ( 'NONE',  ( -92.25000000000056843, -3.200000000000091216, -1.999999999999946265 ) ) ;
#16394=ORIENTED_EDGE ( 'NONE', *, *, #2359, .T. ) ;
#16398=ORIENTED_EDGE ( 'NONE', *, *, #20199, .T. ) ;
#16402=ORIENTED_EDGE ( 'NONE', *, *, #20468, .T. ) ;
#16405=ORIENTED_EDGE ( 'NONE', *, *, #8339, .F. ) ;
#16411=CARTESIAN_POINT ( 'NONE',  ( -55.25320565519145788, 2.700000000000098321, 10.00000000000009237 ) ) ;
#16414=DIRECTION ( 'NONE',  ( 0.7071067811865532349, 0.7071067811865419106, 0.000000000000000000 ) ) ;
#16417=EDGE_CURVE ( 'NONE', #9134, #11001, #8426, .T. ) ;
#16421=DIRECTION ( 'NONE',  ( 1.000000000000000000, -1.550910762415513985E-16, -3.012982189080959477E-32 ) ) ;
#16426=CARTESIAN_POINT ( 'NONE',  ( -89.70000000000059970, 0.5000000000000490719, 1.000000000000000888 ) ) ;
#16432=EDGE_CURVE ( 'NONE', #11081, #16222, #3248, .T. ) ;
#16444=DIRECTION ( 'NONE',  ( 2.013525853228507892E-32, 6.902532920683810383E-31, -1.000000000000000000 ) ) ;
#16456=EDGE_CURVE ( 'NONE', #10432, #12501, #21884, .T. ) ;
#16460=CIRCLE ( 'NONE', #12317, 5.500000000000046185 ) ;
#16470=EDGE_LOOP ( 'NONE', ( #7566, #17217, #12011, #18503 ) ) ;
#16474=DIRECTION ( 'NONE',  ( 1.000000000000000000, -1.550910762415513985E-16, -3.012982189080959477E-32 ) ) ;
#16481=DIRECTION ( 'NONE',  ( 0.9706398123736330597, 1.076300044806638234E-16, 0.2405376366294442736 ) ) ;
#16482=CARTESIAN_POINT ( 'NONE',  ( -6.000000000000019540, -4.800000000000006040, 7.500000000000062172 ) ) ;
#16489=CIRCLE ( 'NONE', #3376, 0.5000000000000029976 ) ;
#16491=ORIENTED_EDGE ( 'NONE', *, *, #2522, .F. ) ;
#16492=ORIENTED_EDGE ( 'NONE', *, *, #1693, .T. ) ;
#16496=ORIENTED_EDGE ( 'NONE', *, *, #1771, .T. ) ;
#16497=DIRECTION ( 'NONE',  ( 0.000000000000000000, -1.000000000000000000, 0.000000000000000000 ) ) ;
#16504=CYLINDRICAL_SURFACE ( 'NONE', #15344, 0.5000000000000037748 ) ;
#16511=DIRECTION ( 'NONE',  ( 2.220446049250313081E-16, -1.000000000000000000, 7.025792437124636392E-31 ) ) ;
#16517=VERTEX_POINT ( 'NONE', #12757 ) ;
#16521=CARTESIAN_POINT ( 'NONE',  ( -45.56568542494951402, -2.108831175456918228, -8.000000000000007105 ) ) ;
#16530=ADVANCED_FACE ( 'NONE', ( #1923 ), #9128, .T. ) ;
#16536=FACE_OUTER_BOUND ( 'NONE', #20310, .T. ) ;
#16539=ORIENTED_EDGE ( 'NONE', *, *, #2092, .T. ) ;
#16551=DIRECTION ( 'NONE',  ( 1.550910762415566494E-16, 1.000000000000000000, -8.135128085091684243E-31 ) ) ;
#16558=AXIS2_PLACEMENT_3D ( 'NONE', #13047, #9755, #939 ) ;
#16588=DIRECTION ( 'NONE',  ( -1.000000000000000000, -1.424116703980846297E-16, 1.095779650622964657E-32 ) ) ;
#16590=AXIS2_PLACEMENT_3D ( 'NONE', #559, #7493, #11350 ) ;
#16596=ORIENTED_EDGE ( 'NONE', *, *, #20495, .T. ) ;
#16598=ORIENTED_EDGE ( 'NONE', *, *, #16692, .T. ) ;
#16606=DIRECTION ( 'NONE',  ( 2.013525853228507892E-32, 6.902532920683810383E-31, -1.000000000000000000 ) ) ;
#16613=CARTESIAN_POINT ( 'NONE',  ( -92.25000000000065370, 5.494493748869900097E-14, -2.000000000000001776 ) ) ;
#16618=FACE_OUTER_BOUND ( 'NONE', #3800, .T. ) ;
#16625=TOROIDAL_SURFACE ( 'NONE', #15927, 2.500000000000003997, 0.5000000000000000000 ) ;
#16632=AXIS2_PLACEMENT_3D ( 'NONE', #21903, #7213, #2018 ) ;
#16634=ORIENTED_EDGE ( 'NONE', *, *, #6783, .F. ) ;
#16636=EDGE_LOOP ( 'NONE', ( #10691, #1801, #22966, #15067 ) ) ;
#16640=DIRECTION ( 'NONE',  ( 2.013525853228507892E-32, 6.902532920683810383E-31, -1.000000000000000000 ) ) ;
#16641=AXIS2_PLACEMENT_3D ( 'NONE', #21997, #5884, #5656 ) ;
#16644=DIRECTION ( 'NONE',  ( -0.7071067811865513475, 0.7071067811865437980, 2.580274238642642345E-14 ) ) ;
#16653=LINE ( 'NONE', #565, #5019 ) ;
#16656=CARTESIAN_POINT ( 'NONE',  ( -50.65685424949273141, 7.200000000000025935, 8.000000000000076383 ) ) ;
#16658=ORIENTED_EDGE ( 'NONE', *, *, #3134, .F. ) ;
#16659=EDGE_CURVE ( 'NONE', #9446, #18130, #12873, .T. ) ;
#16665=CARTESIAN_POINT ( 'NONE',  ( -6.000000000000019540, -7.500000000000007105, 7.500000000000062172 ) ) ;
#16669=DIRECTION ( 'NONE',  ( 1.000000000000000000, 1.065615849528602702E-14, 0.000000000000000000 ) ) ;
#16671=CYLINDRICAL_SURFACE ( 'NONE', #21198, 0.5000000000000025535 ) ;
#16679=AXIS2_PLACEMENT_3D ( 'NONE', #7080, #5538, #18115 ) ;
#16684=EDGE_CURVE ( 'NONE', #14824, #17188, #14748, .T. ) ;
#16685=CARTESIAN_POINT ( 'NONE',  ( -2.700000000000063238, -2.000000000000043521, 8.000000000000076383 ) ) ;
#16692=EDGE_CURVE ( 'NONE', #2652, #4603, #5740, .T. ) ;
#16697=CARTESIAN_POINT ( 'NONE',  ( -43.46238456605047418, 4.919238815542508192, 8.000000000000035527 ) ) ;
#16698=CARTESIAN_POINT ( 'NONE',  ( -45.91923881554273379, -2.462384566050232593, 7.500000000000034639 ) ) ;
#16718=EDGE_CURVE ( 'NONE', #11081, #14890, #7700, .T. ) ;
#16719=VERTEX_POINT ( 'NONE', #22047 ) ;
#16720=VERTEX_POINT ( 'NONE', #2280 ) ;
#16725=ORIENTED_EDGE ( 'NONE', *, *, #18294, .T. ) ;
#16732=LINE ( 'NONE', #2626, #6277 ) ;
#16733=CARTESIAN_POINT ( 'NONE',  ( -95.20000000000065654, -2.700000000000119194, -2.000000000000001776 ) ) ;
#16734=CARTESIAN_POINT ( 'NONE',  ( -65.00000000000044054, -2.700000000000084110, 2.999999999999947153 ) ) ;
#16740=DIRECTION ( 'NONE',  ( -1.550910762415566494E-16, -1.000000000000000000, 8.135128085091684243E-31 ) ) ;
#16747=ORIENTED_EDGE ( 'NONE', *, *, #13692, .T. ) ;
#16753=CARTESIAN_POINT ( 'NONE',  ( -53.99613665484947944, -1.040834085586084257E-13, -13.19342998475045370 ) ) ;
#16765=VECTOR ( 'NONE', #17560, 1000.000000000000114 ) ;
#16792=LINE ( 'NONE', #713, #11945 ) ;
#16800=EDGE_LOOP ( 'NONE', ( #9221, #10882, #20972, #8148 ) ) ;
#16801=ORIENTED_EDGE ( 'NONE', *, *, #20091, .F. ) ;
#16817=CIRCLE ( 'NONE', #21366, 6.000000000000047073 ) ;
#16818=EDGE_CURVE ( 'NONE', #22996, #2097, #15101, .T. ) ;
#16824=DIRECTION ( 'NONE',  ( 1.000000000000000000, 1.479114197289388027E-30, -2.013525853228518840E-32 ) ) ;
#16826=EDGE_CURVE ( 'NONE', #13088, #6327, #6858, .T. ) ;
#16829=VERTEX_POINT ( 'NONE', #6401 ) ;
#16831=AXIS2_PLACEMENT_3D ( 'NONE', #22602, #11538, #9667 ) ;
#16833=ORIENTED_EDGE ( 'NONE', *, *, #20908, .F. ) ;
#16835=VERTEX_POINT ( 'NONE', #1220 ) ;
#16839=ORIENTED_EDGE ( 'NONE', *, *, #10639, .T. ) ;
#16847=CARTESIAN_POINT ( 'NONE',  ( -56.91911807125110556, 1.387778780781445676E-14, -8.333333333333358794 ) ) ;
#16848=DIRECTION ( 'NONE',  ( -2.013525853228507892E-32, -6.902532920683810383E-31, 1.000000000000000000 ) ) ;
#16855=SURFACE_STYLE_USAGE ( .BOTH. , #14984 ) ;
#16857=CARTESIAN_POINT ( 'NONE',  ( -57.28378781035996070, -3.200000000000108979, 8.541666666666781538 ) ) ;
#16868=EDGE_LOOP ( 'NONE', ( #17274, #9396, #2277, #16251 ) ) ;
#16875=CARTESIAN_POINT ( 'NONE',  ( -8.326672684688674053E-14, -2.000000000000029310, 8.000000000000076383 ) ) ;
#16880=PLANE ( 'NONE',  #830 ) ;
#16885=AXIS2_PLACEMENT_3D ( 'NONE', #4039, #18398, #14410 ) ;
#16890=FACE_OUTER_BOUND ( 'NONE', #22850, .T. ) ;
#16892=ORIENTED_EDGE ( 'NONE', *, *, #13695, .T. ) ;
#16895=ORIENTED_EDGE ( 'NONE', *, *, #19140, .T. ) ;
#16902=DIRECTION ( 'NONE',  ( -2.013525853228508439E-32, -6.779273404243028164E-31, 1.000000000000000000 ) ) ;
#16909=CARTESIAN_POINT ( 'NONE',  ( -42.54314575050785407, -4.800000000000037126, -7.500000000000007105 ) ) ;
#16916=CIRCLE ( 'NONE', #17681, 0.5000000000000000000 ) ;
#16920=EDGE_LOOP ( 'NONE', ( #13154, #21057, #5948, #15098 ) ) ;
#16927=DIRECTION ( 'NONE',  ( 0.7071067811865490160, 0.7071067811865460184, 1.565905175853766674E-16 ) ) ;
#16931=DIRECTION ( 'NONE',  ( 1.000000000000000000, 3.144186300207927518E-14, 0.000000000000000000 ) ) ;
#16944=EDGE_CURVE ( 'NONE', #19930, #11087, #498, .T. ) ;
#16945=EDGE_LOOP ( 'NONE', ( #23152, #11550, #13592, #7295 ) ) ;
#16948=ORIENTED_EDGE ( 'NONE', *, *, #3936, .F. ) ;
#16953=EDGE_CURVE ( 'NONE', #13979, #17272, #10944, .T. ) ;
#16960=DIRECTION ( 'NONE',  ( -1.000000000000000000, -6.640738306473676004E-15, -4.078150875473213127E-31 ) ) ;
#16962=AXIS2_PLACEMENT_3D ( 'NONE', #15409, #22597, #8015 ) ;
#16970=EDGE_LOOP ( 'NONE', ( #17707, #22068, #19703, #10458 ) ) ;
#16980=CARTESIAN_POINT ( 'NONE',  ( -66.55000000000046612, -7.593235069856354823E-14, -2.000000000000001776 ) ) ;
#16982=ADVANCED_FACE ( 'NONE', ( #22013 ), #13190, .F. ) ;
#16983=CARTESIAN_POINT ( 'NONE',  ( -57.28378781036000333, 2.700000000000098321, 8.541666666666698049 ) ) ;
#16996=CARTESIAN_POINT ( 'NONE',  ( -42.54314575050785407, -7.500000000000038192, -7.500000000000007105 ) ) ;
#16999=ORIENTED_EDGE ( 'NONE', *, *, #11667, .F. ) ;
#17002=EDGE_CURVE ( 'NONE', #20537, #1136, #18163, .T. ) ;
#17007=EDGE_CURVE ( 'NONE', #9368, #16222, #21157, .T. ) ;
#17009=ORIENTED_EDGE ( 'NONE', *, *, #1237, .F. ) ;
#17021=VECTOR ( 'NONE', #3058, 1000.000000000000000 ) ;
#17023=DIRECTION ( 'NONE',  ( -1.000000000000000000, -1.700709290173333260E-16, 0.000000000000000000 ) ) ;
#17031=CARTESIAN_POINT ( 'NONE',  ( -89.70000000000059970, 0.5000000000000490719, 1.000000000000000888 ) ) ;
#17032=CIRCLE ( 'NONE', #1292, 6.000000000000047073 ) ;
#17041=EDGE_LOOP ( 'NONE', ( #12302, #20254, #8779, #16839 ) ) ;
#17043=LINE ( 'NONE', #9888, #17021 ) ;
#17046=CARTESIAN_POINT ( 'NONE',  ( -0.5000000000000975886, -2.775557561562891351E-14, -7.500000000000007105 ) ) ;
#17047=ORIENTED_EDGE ( 'NONE', *, *, #21203, .T. ) ;
#17049=CARTESIAN_POINT ( 'NONE',  ( -45.37157287525408833, -6.828427124746218269, -8.000000000000062172 ) ) ;
#17054=DIRECTION ( 'NONE',  ( 2.013525853228507892E-32, 6.902532920683810383E-31, -1.000000000000000000 ) ) ;
#17067=VERTEX_POINT ( 'NONE', #3894 ) ;
#17072=ORIENTED_EDGE ( 'NONE', *, *, #10214, .F. ) ;
#17075=FACE_OUTER_BOUND ( 'NONE', #10935, .T. ) ;
#17076=DIRECTION ( 'NONE',  ( 0.7071067811865485719, -0.7071067811865464625, -1.010793663541191485E-16 ) ) ;
#17083=DIRECTION ( 'NONE',  ( 1.000000000000000000, -1.424116703980815236E-16, -2.931272055834072201E-32 ) ) ;
#17093=ORIENTED_EDGE ( 'NONE', *, *, #13838, .F. ) ;
#17096=VECTOR ( 'NONE', #15975, 1000.000000000000000 ) ;
#17098=ORIENTED_EDGE ( 'NONE', *, *, #227, .F. ) ;
#17107=CARTESIAN_POINT ( 'NONE',  ( -6.000000000000102141, 4.799999999999964295, 8.000000000000047962 ) ) ;
#17108=CIRCLE ( 'NONE', #15608, 2.550000000000010481 ) ;
#17110=CARTESIAN_POINT ( 'NONE',  ( -55.05572809000125289, 0.5000000000000143219, -10.00000000000006395 ) ) ;
#17117=ORIENTED_EDGE ( 'NONE', *, *, #18450, .T. ) ;
#17123=ADVANCED_FACE ( 'NONE', ( #18373 ), #4824, .T. ) ;
#17130=DIRECTION ( 'NONE',  ( -1.550910762415566494E-16, -1.000000000000000000, 8.135128085091684243E-31 ) ) ;
#17133=CYLINDRICAL_SURFACE ( 'NONE', #12265, 0.5000000000000028866 ) ;
#17134=CARTESIAN_POINT ( 'NONE',  ( -42.54314575050782565, -4.000000000000034639, -8.000000000000007105 ) ) ;
#17136=CIRCLE ( 'NONE', #7025, 0.5000000000000029976 ) ;
#17137=CARTESIAN_POINT ( 'NONE',  ( -50.65685424949267457, -7.200000000000049916, 7.500000000000047962 ) ) ;
#17140=AXIS2_PLACEMENT_3D ( 'NONE', #16996, #6321, #11835 ) ;
#17148=LINE ( 'NONE', #2931, #2104 ) ;
#17157=AXIS2_PLACEMENT_3D ( 'NONE', #18835, #2711, #22599 ) ;
#17161=CARTESIAN_POINT ( 'NONE',  ( -50.65685424949274562, -0.5000000000001045830, 8.000000000000062172 ) ) ;
#17164=ORIENTED_EDGE ( 'NONE', *, *, #10677, .F. ) ;
#17166=DIRECTION ( 'NONE',  ( 0.2405376366294412205, 0.000000000000000000, -0.9706398123736338368 ) ) ;
#17171=AXIS2_PLACEMENT_3D ( 'NONE', #18457, #7640, #13287 ) ;
#17174=EDGE_CURVE ( 'NONE', #4432, #15682, #12134, .T. ) ;
#17185=EDGE_LOOP ( 'NONE', ( #19395, #10169, #19031, #10121, #19763, #13714, #1525, #3057, #8061, #16031, #11346, #5611 ) ) ;
#17186=ORIENTED_EDGE ( 'NONE', *, *, #6550, .T. ) ;
#17188=VERTEX_POINT ( 'NONE', #13658 ) ;
#17193=AXIS2_PLACEMENT_3D ( 'NONE', #1830, #10658, #21496 ) ;
#17205=DIRECTION ( 'NONE',  ( 1.000000000000000000, 1.424116703980846297E-16, -1.095779650622964657E-32 ) ) ;
#17206=ADVANCED_FACE ( 'NONE', ( #15640 ), #10260, .T. ) ;
#17207=CARTESIAN_POINT ( 'NONE',  ( -64.00000000000045475, 6.245004513516505540E-14, -1.999999999999974021 ) ) ;
#17210=DIRECTION ( 'NONE',  ( -1.000000000000000000, -2.220446049250314067E-16, 5.825996348268307008E-33 ) ) ;
#17212=CIRCLE ( 'NONE', #14962, 0.5000000000000029976 ) ;
#17213=ORIENTED_EDGE ( 'NONE', *, *, #19283, .F. ) ;
#17217=ORIENTED_EDGE ( 'NONE', *, *, #9991, .F. ) ;
#17231=CARTESIAN_POINT ( 'NONE',  ( -50.65685424949262483, -7.200000000000071232, -16.89924331519437928 ) ) ;
#17232=DIRECTION ( 'NONE',  ( 0.9706398123736300620, 1.281898970984135951E-30, 0.2405376366294562085 ) ) ;
#17236=CIRCLE ( 'NONE', #7129, 0.5000000000000028866 ) ;
#17237=CARTESIAN_POINT ( 'NONE',  ( -89.70000000000048601, -2.700000000000084110, 1.000000000000000888 ) ) ;
#17238=DIRECTION ( 'NONE',  ( 1.000000000000000000, 1.424116703980846297E-16, -1.095779650622964657E-32 ) ) ;
#17242=ORIENTED_EDGE ( 'NONE', *, *, #10839, .T. ) ;
#17243=ORIENTED_EDGE ( 'NONE', *, *, #4167, .F. ) ;
#17246=ORIENTED_EDGE ( 'NONE', *, *, #12419, .T. ) ;
#17249=ORIENTED_EDGE ( 'NONE', *, *, #5098, .T. ) ;
#17250=PLANE ( 'NONE',  #4967 ) ;
#17255=FACE_OUTER_BOUND ( 'NONE', #11870, .T. ) ;
#17260=EDGE_CURVE ( 'NONE', #14890, #12565, #9506, .T. ) ;
#17263=LINE ( 'NONE', #4692, #17953 ) ;
#17272=VERTEX_POINT ( 'NONE', #19179 ) ;
#17274=ORIENTED_EDGE ( 'NONE', *, *, #3171, .F. ) ;
#17282=CARTESIAN_POINT ( 'NONE',  ( -6.000000000000116351, 7.499999999999958256, -7.500000000000062172 ) ) ;
#17288=FACE_OUTER_BOUND ( 'NONE', #23245, .T. ) ;
#17289=DIRECTION ( 'NONE',  ( 1.000000000000000000, -6.640738306473671271E-15, -4.480856046118915636E-31 ) ) ;
#17293=EDGE_CURVE ( 'NONE', #20569, #18939, #5425, .T. ) ;
#17302=ORIENTED_EDGE ( 'NONE', *, *, #9672, .T. ) ;
#17305=ADVANCED_FACE ( 'NONE', ( #10702 ), #10474, .T. ) ;
#17313=DIRECTION ( 'NONE',  ( 1.000000000000000000, 0.000000000000000000, 0.000000000000000000 ) ) ;
#17316=CARTESIAN_POINT ( 'NONE',  ( -47.47487373415322764, -4.018019484660590557, 8.000000000000145661 ) ) ;
#17328=ORIENTED_EDGE ( 'NONE', *, *, #6054, .F. ) ;
#17334=CYLINDRICAL_SURFACE ( 'NONE', #4676, 0.5000000000000004441 ) ;
#17336=AXIS2_PLACEMENT_3D ( 'NONE', #22219, #578, #9984 ) ;
#17337=DIRECTION ( 'NONE',  ( 2.013525853228507892E-32, 6.902532920683810383E-31, -1.000000000000000000 ) ) ;
#17348=PLANE ( 'NONE',  #2581 ) ;
#17356=VECTOR ( 'NONE', #16640, 1000.000000000000000 ) ;
#17358=ORIENTED_EDGE ( 'NONE', *, *, #22199, .T. ) ;
#17359=ORIENTED_EDGE ( 'NONE', *, *, #21959, .T. ) ;
#17362=CARTESIAN_POINT ( 'NONE',  ( -42.54314575050781144, -3.999999999999996447, -16.42537846091818210 ) ) ;
#17368=CARTESIAN_POINT ( 'NONE',  ( -52.60445557845689990, 9.020562075079396891E-14, 15.85914177512520773 ) ) ;
#17370=VECTOR ( 'NONE', #12043, 1000.000000000000000 ) ;
#17375=AXIS2_PLACEMENT_3D ( 'NONE', #4786, #4893, #19492 ) ;
#17381=ADVANCED_FACE ( 'NONE', ( #18006 ), #18919, .T. ) ;
#17387=AXIS2_PLACEMENT_3D ( 'NONE', #18508, #4821, #6169 ) ;
#17390=CIRCLE ( 'NONE', #6143, 2.550000000000010481 ) ;
#17391=ORIENTED_EDGE ( 'NONE', *, *, #18713, .F. ) ;
#17406=CIRCLE ( 'NONE', #6899, 0.5000000000000004441 ) ;
#17407=FACE_OUTER_BOUND ( 'NONE', #22119, .T. ) ;
#17412=DIRECTION ( 'NONE',  ( 0.000000000000000000, 0.000000000000000000, 1.000000000000000000 ) ) ;
#17414=ORIENTED_EDGE ( 'NONE', *, *, #426, .T. ) ;
#17416=EDGE_CURVE ( 'NONE', #9299, #18640, #12151, .T. ) ;
#17417=ORIENTED_EDGE ( 'NONE', *, *, #5225, .F. ) ;
#17423=ORIENTED_EDGE ( 'NONE', *, *, #19165, .T. ) ;
#17426=LINE ( 'NONE', #8496, #6512 ) ;
#17427=VECTOR ( 'NONE', #12513, 1000.000000000000000 ) ;
#17432=DIRECTION ( 'NONE',  ( -1.000000000000000000, -2.220446049250307904E-16, 0.000000000000000000 ) ) ;
#17439=DIRECTION ( 'NONE',  ( -1.000000000000000000, 1.700709290173333260E-16, 0.000000000000000000 ) ) ;
#17444=VECTOR ( 'NONE', #3197, 1000.000000000000000 ) ;
#17454=EDGE_LOOP ( 'NONE', ( #6813, #5633, #14253, #8236 ) ) ;
#17457=EDGE_LOOP ( 'NONE', ( #5588, #4677, #9596, #7966, #13236, #9589, #17047, #11659, #19808, #8265, #9017, #12416 ) ) ;
#17459=AXIS2_PLACEMENT_3D ( 'NONE', #8129, #11765, #20851 ) ;
#17471=DIRECTION ( 'NONE',  ( 1.550910762415566494E-16, 1.000000000000000000, -8.135128085091684243E-31 ) ) ;
#17492=DIRECTION ( 'NONE',  ( 1.000000000000000000, 3.026128730315075503E-14, 0.000000000000000000 ) ) ;
#17508=ORIENTED_EDGE ( 'NONE', *, *, #11822, .F. ) ;
#17512=ORIENTED_EDGE ( 'NONE', *, *, #21013, .F. ) ;
#17514=CIRCLE ( 'NONE', #17140, 0.5000000000000029976 ) ;
#17516=DIRECTION ( 'NONE',  ( 1.000000000000000000, 2.282530889443153710E-16, 8.673617379883983210E-16 ) ) ;
#17523=DIRECTION ( 'NONE',  ( -1.000000000000000000, 1.065615849528602702E-14, 0.000000000000000000 ) ) ;
#17528=PLANE ( 'NONE',  #7829 ) ;
#17530=VERTEX_POINT ( 'NONE', #12700 ) ;
#17534=ORIENTED_EDGE ( 'NONE', *, *, #10358, .T. ) ;
#17537=AXIS2_PLACEMENT_3D ( 'NONE', #12559, #5278, #19748 ) ;
#17549=DIRECTION ( 'NONE',  ( -0.7071067811865535679, 0.7071067811865414665, 0.000000000000000000 ) ) ;
#17551=CARTESIAN_POINT ( 'NONE',  ( -57.28378781035998912, -0.5000000000000281997, 8.541666666666767327 ) ) ;
#17556=CARTESIAN_POINT ( 'NONE',  ( -6.000000000000074607, -7.500000000000027534, -7.500000000000034639 ) ) ;
#17560=DIRECTION ( 'NONE',  ( 0.9878135252003127365, 2.193386639427060722E-16, -0.1556420233463029767 ) ) ;
#17568=CIRCLE ( 'NONE', #17193, 0.5000000000000014433 ) ;
#17571=ORIENTED_EDGE ( 'NONE', *, *, #9598, .F. ) ;
#17576=CIRCLE ( 'NONE', #310, 5.500000000000032863 ) ;
#17577=DIRECTION ( 'NONE',  ( -0.7071067811865507924, -0.7071067811865444641, -2.121016688166342479E-16 ) ) ;
#17578=EDGE_CURVE ( 'NONE', #21118, #18025, #8536, .T. ) ;
#17579=ORIENTED_EDGE ( 'NONE', *, *, #183, .T. ) ;
#17580=DIRECTION ( 'NONE',  ( -0.7071067811865490160, -0.7071067811865460184, -1.565905175853766674E-16 ) ) ;
#17588=ADVANCED_FACE ( 'NONE', ( #4997 ), #1588, .F. ) ;
#17590=DIRECTION ( 'NONE',  ( 1.000000000000000000, 1.479114197289387852E-30, -2.013525853228518840E-32 ) ) ;
#17592=DIRECTION ( 'NONE',  ( 1.000000000000000000, 1.479114197289388027E-30, -2.013525853228518840E-32 ) ) ;
#17593=VECTOR ( 'NONE', #19740, 1000.000000000000000 ) ;
#17601=CIRCLE ( 'NONE', #4445, 1.300000000000009592 ) ;
#17607=DIRECTION ( 'NONE',  ( 2.013525853228507892E-32, 6.902532920683810383E-31, -1.000000000000000000 ) ) ;
#17608=CARTESIAN_POINT ( 'NONE',  ( -45.37157287525420202, 6.828427124746169419, 7.500000000000089706 ) ) ;
#17612=DIRECTION ( 'NONE',  ( 0.9706398123736329486, 2.155253336630096955E-16, 0.2405376366294442458 ) ) ;
#17614=LINE ( 'NONE', #1506, #4575 ) ;
#17616=TOROIDAL_SURFACE ( 'NONE', #13124, 2.500000000000002220, 0.5000000000000000000 ) ;
#17617=DIRECTION ( 'NONE',  ( -1.000000000000000000, 3.742046355321372466E-14, 0.000000000000000000 ) ) ;
#17630=ORIENTED_EDGE ( 'NONE', *, *, #16826, .F. ) ;
#17635=CARTESIAN_POINT ( 'NONE',  ( -45.56568542494951402, 2.108831175456883589, 8.000000000000035527 ) ) ;
#17651=ORIENTED_EDGE ( 'NONE', *, *, #7216, .T. ) ;
#17666=CARTESIAN_POINT ( 'NONE',  ( -90.63385214007838897, -7.632783294297951215E-14, -7.926881151201908615 ) ) ;
#17674=CARTESIAN_POINT ( 'NONE',  ( -2.700000000000035705, 7.199999999999977085, -7.500000000000007105 ) ) ;
#17675=DIRECTION ( 'NONE',  ( 2.013525853228507892E-32, 6.902532920683810383E-31, -1.000000000000000000 ) ) ;
#17676=CARTESIAN_POINT ( 'NONE',  ( -55.05572809000122447, -2.700000000000125855, -10.00000000000006395 ) ) ;
#17679=VERTEX_POINT ( 'NONE', #190 ) ;
#17681=AXIS2_PLACEMENT_3D ( 'NONE', #18601, #2591, #4470 ) ;
#17684=ORIENTED_EDGE ( 'NONE', *, *, #11622, .F. ) ;
#17691=EDGE_CURVE ( 'NONE', #7127, #20569, #6159, .T. ) ;
#17693=DIRECTION ( 'NONE',  ( -2.220446049250313081E-16, 1.000000000000000000, -7.025792437124636392E-31 ) ) ;
#17696=CARTESIAN_POINT ( 'NONE',  ( -50.65685424949280247, 2.700000000000021938, 8.000000000000090594 ) ) ;
#17703=DIRECTION ( 'NONE',  ( 0.7071067811865517916, 0.7071067811865431318, 4.556821512286124754E-17 ) ) ;
#17705=DIRECTION ( 'NONE',  ( -2.013525853228507892E-32, -6.902532920683810383E-31, 1.000000000000000000 ) ) ;
#17707=ORIENTED_EDGE ( 'NONE', *, *, #6119, .T. ) ;
#17710=CARTESIAN_POINT ( 'NONE',  ( -55.05572809000125289, 1.387778780781445676E-14, -10.00000000000006395 ) ) ;
#17713=EDGE_CURVE ( 'NONE', #3480, #19838, #9116, .T. ) ;
#17721=ORIENTED_EDGE ( 'NONE', *, *, #1374, .T. ) ;
#17738=DIRECTION ( 'NONE',  ( 1.000000000000000000, 2.168404344970992105E-16, 1.734723475976793684E-15 ) ) ;
#17749=FACE_OUTER_BOUND ( 'NONE', #5110, .T. ) ;
#17750=VERTEX_POINT ( 'NONE', #11329 ) ;
#17751=ORIENTED_EDGE ( 'NONE', *, *, #2359, .F. ) ;
#17756=CARTESIAN_POINT ( 'NONE',  ( -89.70000000000057128, -9.020562075079396891E-14, -2.000000000000001776 ) ) ;
#17767=DIRECTION ( 'NONE',  ( 2.013525853228507892E-32, 6.902532920683810383E-31, -1.000000000000000000 ) ) ;
#17772=CARTESIAN_POINT ( 'NONE',  ( -55.25320565519152893, 2.700000000000104983, 8.000000000000035527 ) ) ;
#17781=ORIENTED_EDGE ( 'NONE', *, *, #8838, .T. ) ;
#17787=ORIENTED_EDGE ( 'NONE', *, *, #196, .T. ) ;
#17790=CARTESIAN_POINT ( 'NONE',  ( -61.45000000000046469, 6.301625887772388776E-14, -1.999999999999973577 ) ) ;
#17799=DIRECTION ( 'NONE',  ( 0.7071067811865457964, 0.7071067811865492381, 0.000000000000000000 ) ) ;
#17815=ORIENTED_EDGE ( 'NONE', *, *, #22926, .F. ) ;
#17826=FACE_OUTER_BOUND ( 'NONE', #3660, .T. ) ;
#17829=VECTOR ( 'NONE', #5451, 1000.000000000000114 ) ;
#17841=DIRECTION ( 'NONE',  ( -2.013525853228508439E-32, -6.779273404243028164E-31, 1.000000000000000000 ) ) ;
#17845=CIRCLE ( 'NONE', #8457, 6.000000000000047073 ) ;
#17847=VECTOR ( 'NONE', #1333, 1000.000000000000000 ) ;
#17853=CYLINDRICAL_SURFACE ( 'NONE', #15085, 0.5000000000000036637 ) ;
#17854=EDGE_CURVE ( 'NONE', #22258, #22523, #21584, .T. ) ;
#17862=VECTOR ( 'NONE', #4576, 1000.000000000000000 ) ;
#17885=DIRECTION ( 'NONE',  ( 1.000000000000000000, -1.424116703980815236E-16, -2.931272055834072201E-32 ) ) ;
#17886=CIRCLE ( 'NONE', #14134, 6.000000000000047073 ) ;
#17897=VECTOR ( 'NONE', #20335, 1000.000000000000000 ) ;
#17901=VERTEX_POINT ( 'NONE', #17316 ) ;
#17910=EDGE_CURVE ( 'NONE', #5689, #9100, #6548, .T. ) ;
#17913=CARTESIAN_POINT ( 'NONE',  ( -64.00000000000045475, -7.632783294297951215E-14, -2.000000000000001776 ) ) ;
#17919=EDGE_CURVE ( 'NONE', #16028, #10146, #19208, .T. ) ;
#17921=FACE_OUTER_BOUND ( 'NONE', #16920, .T. ) ;
#17925=ORIENTED_EDGE ( 'NONE', *, *, #8112, .F. ) ;
#17937=CIRCLE ( 'NONE', #13044, 2.500000000000015987 ) ;
#17943=DIRECTION ( 'NONE',  ( 1.000000000000000000, 0.000000000000000000, 0.000000000000000000 ) ) ;
#17947=CIRCLE ( 'NONE', #20585, 2.000000000000015543 ) ;
#17953=VECTOR ( 'NONE', #8104, 1000.000000000000114 ) ;
#17960=ORIENTED_EDGE ( 'NONE', *, *, #3507, .F. ) ;
#17962=CIRCLE ( 'NONE', #18321, 4.000000000000023981 ) ;
#17963=ADVANCED_FACE ( 'NONE', ( #3226 ), #4741, .F. ) ;
#17965=ORIENTED_EDGE ( 'NONE', *, *, #14260, .T. ) ;
#17970=DIRECTION ( 'NONE',  ( -2.013525853228507892E-32, -6.902532920683810383E-31, 1.000000000000000000 ) ) ;
#17977=CARTESIAN_POINT ( 'NONE',  ( -3.200000000000049916, 5.299999999999957190, -7.500000000000034639 ) ) ;
#17983=LINE ( 'NONE', #1848, #10646 ) ;
#17990=EDGE_CURVE ( 'NONE', #4065, #9788, #18559, .T. ) ;
#18003=LINE ( 'NONE', #23187, #9900 ) ;
#18006=FACE_OUTER_BOUND ( 'NONE', #10284, .T. ) ;
#18010=DIRECTION ( 'NONE',  ( -0.9706398123736330597, 1.505375731439247434E-16, -0.2405376366294442736 ) ) ;
#18023=ORIENTED_EDGE ( 'NONE', *, *, #13997, .F. ) ;
#18025=VERTEX_POINT ( 'NONE', #14271 ) ;
#18033=DIRECTION ( 'NONE',  ( 2.220446049250313081E-16, -1.000000000000000000, 7.025792437124636392E-31 ) ) ;
#18049=UNCERTAINTY_MEASURE_WITH_UNIT (LENGTH_MEASURE( 1.000000000000000082E-05 ), #441, 'distance_accuracy_value', 'NONE');
#18053=ORIENTED_EDGE ( 'NONE', *, *, #21203, .F. ) ;
#18054=ORIENTED_EDGE ( 'NONE', *, *, #6951, .F. ) ;
#18055=CIRCLE ( 'NONE', #15023, 2.000000000000015543 ) ;
#18061=CARTESIAN_POINT ( 'NONE',  ( -95.20000000000061391, -9.714451465470119729E-14, 1.000000000000028644 ) ) ;
#18064=LINE ( 'NONE', #13109, #14767 ) ;
#18065=CYLINDRICAL_SURFACE ( 'NONE', #10847, 0.5000000000000012212 ) ;
#18078=ORIENTED_EDGE ( 'NONE', *, *, #4211, .F. ) ;
#18082=DIRECTION ( 'NONE',  ( -1.387778780781445676E-14, -1.000000000000000000, 0.000000000000000000 ) ) ;
#18084=CARTESIAN_POINT ( 'NONE',  ( -1.110223024625156540E-13, -1.999999999999988010, 7.500000000000020428 ) ) ;
#18085=FACE_OUTER_BOUND ( 'NONE', #8605, .T. ) ;
#18087=CARTESIAN_POINT ( 'NONE',  ( -55.05572809000126711, 1.387778780781445676E-14, -7.500000000000034639 ) ) ;
#18096=TOROIDAL_SURFACE ( 'NONE', #21105, 2.500000000000003997, 0.5000000000000000000 ) ;
#18105=PLANE ( 'NONE',  #22531 ) ;
#18108=AXIS2_PLACEMENT_3D ( 'NONE', #19736, #21510, #5619 ) ;
#18115=DIRECTION ( 'NONE',  ( -0.7071067811865449082, 0.7071067811865501263, 0.000000000000000000 ) ) ;
#18116=CARTESIAN_POINT ( 'NONE',  ( -95.20000000000065654, 0.5000000000000073275, 8.000000000000076383 ) ) ;
#18117=DIRECTION ( 'NONE',  ( 1.000000000000000000, 1.734723475976796001E-16, 0.000000000000000000 ) ) ;
#18118=AXIS2_PLACEMENT_3D ( 'NONE', #20986, #22517, #14037 ) ;
#18124=ORIENTED_EDGE ( 'NONE', *, *, #21755, .T. ) ;
#18130=VERTEX_POINT ( 'NONE', #16017 ) ;
#18142=DIRECTION ( 'NONE',  ( -1.550910762415566494E-16, -1.000000000000000000, 8.135128085091684243E-31 ) ) ;
#18152=CARTESIAN_POINT ( 'NONE',  ( -64.00000000000045475, 6.245004513516505540E-14, -1.999999999999974021 ) ) ;
#18158=ORIENTED_EDGE ( 'NONE', *, *, #14592, .F. ) ;
#18163=CIRCLE ( 'NONE', #8388, 0.5000000000000028866 ) ;
#18169=AXIS2_PLACEMENT_3D ( 'NONE', #3339, #14150, #3445 ) ;
#18173=EDGE_LOOP ( 'NONE', ( #14509, #12180, #4367, #3714 ) ) ;
#18186=CIRCLE ( 'NONE', #6916, 3.300000000000019806 ) ;
#18190=CIRCLE ( 'NONE', #11030, 2.550000000000010481 ) ;
#18196=EDGE_LOOP ( 'NONE', ( #2994, #17751, #11040, #12158 ) ) ;
#18197=VERTEX_POINT ( 'NONE', #6024 ) ;
#18204=CYLINDRICAL_SURFACE ( 'NONE', #21532, 6.000000000000000000 ) ;
#18210=CYLINDRICAL_SURFACE ( 'NONE', #2111, 0.5000000000000004441 ) ;
#18215=EDGE_CURVE ( 'NONE', #4366, #13948, #3900, .T. ) ;
#18236=PLANE ( 'NONE',  #553 ) ;
#18285=CARTESIAN_POINT ( 'NONE',  ( -9.714451465470119729E-14, 1.999999999999890754, 8.000000000000090594 ) ) ;
#18288=LINE ( 'NONE', #18515, #3341 ) ;
#18289=CARTESIAN_POINT ( 'NONE',  ( -66.55000000000039506, -3.200000000000081002, -2.000000000000029310 ) ) ;
#18292=ORIENTED_EDGE ( 'NONE', *, *, #333, .F. ) ;
#18294=EDGE_CURVE ( 'NONE', #13948, #13984, #2709, .T. ) ;
#18300=ORIENTED_EDGE ( 'NONE', *, *, #13863, .T. ) ;
#18312=LINE ( 'NONE', #2190, #3466 ) ;
#18321=AXIS2_PLACEMENT_3D ( 'NONE', #21429, #1756, #12808 ) ;
#18325=SURFACE_SIDE_STYLE ('',( #11479 ) ) ;
#18326=CARTESIAN_POINT ( 'NONE',  ( -65.55642023346347003, -8.326672684688674053E-14, -11.87813525200320797 ) ) ;
#18329=AXIS2_PLACEMENT_3D ( 'NONE', #20828, #3727, #6929 ) ;
#18333=CARTESIAN_POINT ( 'NONE',  ( -56.91911807125098477, -3.200000000000108979, -8.333333333333413862 ) ) ;
#18336=DIRECTION ( 'NONE',  ( 1.000000000000000000, 1.479114197289387852E-30, -2.013525853228518840E-32 ) ) ;
#18339=DIRECTION ( 'NONE',  ( 1.550910762415566494E-16, 1.000000000000000000, -8.135128085091684243E-31 ) ) ;
#18356=ADVANCED_FACE ( 'NONE', ( #17288 ), #16625, .T. ) ;
#18357=AXIS2_PLACEMENT_3D ( 'NONE', #21976, #18664, #798 ) ;
#18362=ORIENTED_EDGE ( 'NONE', *, *, #9240, .F. ) ;
#18371=VECTOR ( 'NONE', #15638, 1000.000000000000114 ) ;
#18373=FACE_OUTER_BOUND ( 'NONE', #15755, .T. ) ;
#18383=LINE ( 'NONE', #9440, #18695 ) ;
#18390=ORIENTED_EDGE ( 'NONE', *, *, #472, .F. ) ;
#18397=CARTESIAN_POINT ( 'NONE',  ( -45.01801948466080461, -6.474873734152955862, 7.500000000000062172 ) ) ;
#18398=DIRECTION ( 'NONE',  ( 1.550910762415566494E-16, 1.000000000000000000, -8.135128085091684243E-31 ) ) ;
#18424=LINE ( 'NONE', #2191, #5745 ) ;
#18425=DIRECTION ( 'NONE',  ( -0.7071067811865491270, -0.7071067811865461294, -1.565905175853767167E-16 ) ) ;
#18426=VECTOR ( 'NONE', #8617, 1000.000000000000114 ) ;
#18433=CARTESIAN_POINT ( 'NONE',  ( -50.65685424949274562, -3.200000000000091660, 8.000000000000062172 ) ) ;
#18434=ADVANCED_FACE ( 'NONE', ( #22721 ), #6718, .T. ) ;
#18436=FACE_OUTER_BOUND ( 'NONE', #6589, .T. ) ;
#18439=EDGE_CURVE ( 'NONE', #1775, #5689, #11805, .T. ) ;
#18447=EDGE_CURVE ( 'NONE', #19838, #7684, #23193, .T. ) ;
#18450=EDGE_CURVE ( 'NONE', #1694, #5384, #15508, .T. ) ;
#18457=CARTESIAN_POINT ( 'NONE',  ( -42.54314575050785407, -4.000000000000021316, 8.000000000000007105 ) ) ;
#18458=CIRCLE ( 'NONE', #8318, 2.800000000000017586 ) ;
#18466=EDGE_LOOP ( 'NONE', ( #13066, #22212, #20098, #12694 ) ) ;
#18473=CARTESIAN_POINT ( 'NONE',  ( -43.10883117545713361, -4.565685424949256443, -7.500000000000007105 ) ) ;
#18478=DIRECTION ( 'NONE',  ( -1.000000000000000000, -6.938893903907186568E-15, 0.000000000000000000 ) ) ;
#18479=CYLINDRICAL_SURFACE ( 'NONE', #20192, 0.5000000000000000000 ) ;
#18486=CARTESIAN_POINT ( 'NONE',  ( -6.866595637047972822, -4.163336342344337027E-14, 27.70872448147272848 ) ) ;
#18491=AXIS2_PLACEMENT_3D ( 'NONE', #3395, #5147, #17492 ) ;
#18497=ORIENTED_EDGE ( 'NONE', *, *, #16274, .F. ) ;
#18503=ORIENTED_EDGE ( 'NONE', *, *, #3625, .F. ) ;
#18506=VECTOR ( 'NONE', #20055, 1000.000000000000000 ) ;
#18508=CARTESIAN_POINT ( 'NONE',  ( -42.54314575050793934, -4.000000000000021316, 7.500000000000062172 ) ) ;
#18512=DIRECTION ( 'NONE',  ( 1.000000000000000000, 1.479114197289388027E-30, -2.013525853228518840E-32 ) ) ;
#18513=AXIS2_PLACEMENT_3D ( 'NONE', #7397, #20331, #14908 ) ;
#18515=CARTESIAN_POINT ( 'NONE',  ( -6.000000000000088818, -7.500000000000007105, 8.000000000000062172 ) ) ;
#18519=FACE_OUTER_BOUND ( 'NONE', #6160, .T. ) ;
#18523=CARTESIAN_POINT ( 'NONE',  ( -55.05572809000125289, 2.700000000000021938, -10.00000000000006395 ) ) ;
#18525=ORIENTED_EDGE ( 'NONE', *, *, #21283, .F. ) ;
#18532=ORIENTED_EDGE ( 'NONE', *, *, #6081, .T. ) ;
#18533=EDGE_CURVE ( 'NONE', #21802, #6614, #5185, .T. ) ;
#18534=EDGE_LOOP ( 'NONE', ( #21028, #13520, #13159, #1719 ) ) ;
#18540=DIRECTION ( 'NONE',  ( -1.550910762415566494E-16, -1.000000000000000000, 8.135128085091684243E-31 ) ) ;
#18559=CIRCLE ( 'NONE', #19315, 2.550000000000010481 ) ;
#18570=EDGE_CURVE ( 'NONE', #17901, #20601, #20239, .T. ) ;
#18571=FACE_OUTER_BOUND ( 'NONE', #14972, .T. ) ;
#18579=TOROIDAL_SURFACE ( 'NONE', #1304, 2.500000000000002220, 0.5000000000000000000 ) ;
#18582=CYLINDRICAL_SURFACE ( 'NONE', #16641, 0.5000000000000028866 ) ;
#18587=ORIENTED_EDGE ( 'NONE', *, *, #7419, .F. ) ;
#18589=ADVANCED_FACE ( 'NONE', ( #9635 ), #18236, .T. ) ;
#18591=CIRCLE ( 'NONE', #9953, 2.500000000000015987 ) ;
#18593=ORIENTED_EDGE ( 'NONE', *, *, #8232, .T. ) ;
#18594=CIRCLE ( 'NONE', #8459, 0.5000000000000029976 ) ;
#18598=DIRECTION ( 'NONE',  ( -1.000000000000000000, 1.550910762415526064E-16, 0.000000000000000000 ) ) ;
#18601=CARTESIAN_POINT ( 'NONE',  ( -50.65685424949277404, -0.5000000000000905942, -7.500000000000062172 ) ) ;
#18602=ADVANCED_FACE ( 'NONE', ( #20345 ), #18582, .T. ) ;
#18603=CARTESIAN_POINT ( 'NONE',  ( -67.28510754798011817, -2.700000000000125855, 12.22107821754960000 ) ) ;
#18613=CARTESIAN_POINT ( 'NONE',  ( -55.05572809000123868, -1.040834085586084257E-13, -7.500000000000062172 ) ) ;
#18618=ORIENTED_EDGE ( 'NONE', *, *, #1770, .T. ) ;
#18619=EDGE_LOOP ( 'NONE', ( #21525, #2346, #9949, #10571 ) ) ;
#18627=DIRECTION ( 'NONE',  ( 1.000000000000000000, 0.000000000000000000, 0.000000000000000000 ) ) ;
#18636=DIRECTION ( 'NONE',  ( 1.000000000000000000, 1.734723475976796001E-16, 0.000000000000000000 ) ) ;
#18638=VERTEX_POINT ( 'NONE', #4327 ) ;
#18640=VERTEX_POINT ( 'NONE', #11392 ) ;
#18652=EDGE_CURVE ( 'NONE', #5077, #7485, #21878, .T. ) ;
#18653=CARTESIAN_POINT ( 'NONE',  ( -42.54314575050795355, 3.999999999999996447, -7.500000000000007105 ) ) ;
#18654=FACE_OUTER_BOUND ( 'NONE', #19814, .T. ) ;
#18660=CARTESIAN_POINT ( 'NONE',  ( -3.200000000000036149, -2.000000000000043521, 8.000000000000047962 ) ) ;
#18662=EDGE_CURVE ( 'NONE', #11952, #4887, #8227, .T. ) ;
#18663=( NAMED_UNIT ( * ) PLANE_ANGLE_UNIT ( ) SI_UNIT ( $, .RADIAN. ) );
#18664=DIRECTION ( 'NONE',  ( 2.013525853228518840E-32, -6.902532920683810383E-31, 1.000000000000000000 ) ) ;
#18667=ORIENTED_EDGE ( 'NONE', *, *, #6081, .F. ) ;
#18669=VERTEX_POINT ( 'NONE', #6692 ) ;
#18670=ORIENTED_EDGE ( 'NONE', *, *, #4036, .F. ) ;
#18686=CARTESIAN_POINT ( 'NONE',  ( -50.65685424949267457, -7.200000000000071232, -8.000000000000007105 ) ) ;
#18695=VECTOR ( 'NONE', #16588, 1000.000000000000000 ) ;
#18702=ORIENTED_EDGE ( 'NONE', *, *, #12459, .F. ) ;
#18703=ORIENTED_EDGE ( 'NONE', *, *, #15785, .F. ) ;
#18710=CARTESIAN_POINT ( 'NONE',  ( -89.70000000000059970, 2.700000000000056577, 1.000000000000000888 ) ) ;
#18713=EDGE_CURVE ( 'NONE', #15682, #11574, #16258, .T. ) ;
#18721=DIRECTION ( 'NONE',  ( 1.000000000000000000, -1.389842848855773367E-62, 2.013525853228507892E-32 ) ) ;
#18728=ADVANCED_FACE ( 'NONE', ( #1289 ), #18812, .F. ) ;
#18737=FACE_OUTER_BOUND ( 'NONE', #18619, .T. ) ;
#18742=DIRECTION ( 'NONE',  ( -2.220446049250313081E-16, 1.000000000000000000, -7.025792437124636392E-31 ) ) ;
#18746=CARTESIAN_POINT ( 'NONE',  ( -95.70000000000058549, -2.700000000000119194, 1.000000000000014655 ) ) ;
#18749=PLANE ( 'NONE',  #3876 ) ;
#18752=DIRECTION ( 'NONE',  ( -1.000000000000000000, 1.550910762415510534E-16, 0.000000000000000000 ) ) ;
#18755=CARTESIAN_POINT ( 'NONE',  ( -64.00000000000045475, 2.700000000000056577, -1.999999999999974021 ) ) ;
#18761=AXIS2_PLACEMENT_3D ( 'NONE', #7479, #16511, #4162 ) ;
#18762=EDGE_CURVE ( 'NONE', #4432, #14457, #7269, .T. ) ;
#18768=ORIENTED_EDGE ( 'NONE', *, *, #8112, .T. ) ;
#18778=DIRECTION ( 'NONE',  ( -0.7071067811865232589, 0.7071067811865717756, 0.000000000000000000 ) ) ;
#18782=VECTOR ( 'NONE', #17076, 1000.000000000000114 ) ;
#18801=CIRCLE ( 'NONE', #13561, 0.4999999999999994449 ) ;
#18804=DIRECTION ( 'NONE',  ( 2.013525853228507892E-32, 6.902532920683810383E-31, -1.000000000000000000 ) ) ;
#18807=CARTESIAN_POINT ( 'NONE',  ( -95.20000000000065654, 2.700000000000014833, 8.000000000000076383 ) ) ;
#18811=DIRECTION ( 'NONE',  ( 1.000000000000000000, 4.264528545109623427E-14, 0.000000000000000000 ) ) ;
#18812=PLANE ( 'NONE',  #1274 ) ;
#18814=LINE ( 'NONE', #3513, #11121 ) ;
#18815=LINE ( 'NONE', #13757, #2179 ) ;
#18829=CARTESIAN_POINT ( 'NONE',  ( -3.200000000000091660, 1.999999999999980904, -8.000000000000035527 ) ) ;
#18834=DIRECTION ( 'NONE',  ( 1.000000000000000000, -1.550910762415513985E-16, -3.012982189080959477E-32 ) ) ;
#18835=CARTESIAN_POINT ( 'NONE',  ( -6.000000000000088818, -2.000000000000043521, -7.500000000000007105 ) ) ;
#18838=CARTESIAN_POINT ( 'NONE',  ( -6.000000000000074607, -5.300000000000027356, -7.500000000000034639 ) ) ;
#18842=EDGE_LOOP ( 'NONE', ( #15197, #9066, #16634, #7655 ) ) ;
#18848=DIRECTION ( 'NONE',  ( -1.550910762415566494E-16, -1.000000000000000000, 8.135128085091684243E-31 ) ) ;
#18849=EDGE_CURVE ( 'NONE', #22937, #9917, #105, .T. ) ;
#18858=DIRECTION ( 'NONE',  ( -1.939787525279694947E-32, 6.902532920683810383E-31, -1.000000000000000000 ) ) ;
#18866=DIRECTION ( 'NONE',  ( -1.000000000000000000, -2.220446049250301001E-16, 0.000000000000000000 ) ) ;
#18867=CARTESIAN_POINT ( 'NONE',  ( -55.05572809000126711, 3.200000000000022382, -7.500000000000034639 ) ) ;
#18869=CARTESIAN_POINT ( 'NONE',  ( -47.47487373415330580, 4.018019484660594109, -8.000000000000062172 ) ) ;
#18875=EDGE_CURVE ( 'NONE', #22258, #21644, #3137, .T. ) ;
#18878=EDGE_CURVE ( 'NONE', #17901, #21212, #19507, .T. ) ;
#18886=CARTESIAN_POINT ( 'NONE',  ( -50.65685424949270299, 7.200000000000025935, 7.500000000000062172 ) ) ;
#18900=PLANE ( 'NONE',  #20636 ) ;
#18914=VERTEX_POINT ( 'NONE', #19747 ) ;
#18916=CARTESIAN_POINT ( 'NONE',  ( -89.70000000000054285, -0.5000000000000628386, 1.000000000000000888 ) ) ;
#18919=TOROIDAL_SURFACE ( 'NONE', #19673, 5.500000000000000000, 0.5000000000000000000 ) ;
#18928=CARTESIAN_POINT ( 'NONE',  ( -50.65685424949281668, 2.700000000000021938, -7.500000000000089706 ) ) ;
#18929=EDGE_CURVE ( 'NONE', #14402, #13088, #17983, .T. ) ;
#18939=VERTEX_POINT ( 'NONE', #3168 ) ;
#18952=CARTESIAN_POINT ( 'NONE',  ( -52.60445557845680753, -0.5000000000000281997, 15.85914177512520773 ) ) ;
#18962=DIRECTION ( 'NONE',  ( 1.000000000000000000, 2.220446049250314067E-16, -5.825996348268307008E-33 ) ) ;
#18963=DIRECTION ( 'NONE',  ( -2.220446049250313081E-16, 1.000000000000000000, -7.025792437124636392E-31 ) ) ;
#18970=EDGE_LOOP ( 'NONE', ( #19307, #3820, #9673, #6537 ) ) ;
#18980=CARTESIAN_POINT ( 'NONE',  ( -50.65685424949274562, -1.040834085586084257E-13, 8.000000000000062172 ) ) ;
#18984=CYLINDRICAL_SURFACE ( 'NONE', #13306, 0.5000000000000004441 ) ;
#18993=CYLINDRICAL_SURFACE ( 'NONE', #10400, 0.5000000000000000000 ) ;
#19004=EDGE_CURVE ( 'NONE', #13876, #19780, #9612, .T. ) ;
#19005=ORIENTED_EDGE ( 'NONE', *, *, #3392, .T. ) ;
#19006=DIRECTION ( 'NONE',  ( -0.9878135252003127365, 1.532010627492774434E-16, 0.1556420233463029767 ) ) ;
#19009=EDGE_LOOP ( 'NONE', ( #5285, #22603, #15064, #1384 ) ) ;
#19015=CARTESIAN_POINT ( 'NONE',  ( -91.02295700146262902, 2.700000000000014833, 6.338518968055040226 ) ) ;
#19020=DIRECTION ( 'NONE',  ( -2.220446049250313081E-16, 1.000000000000000000, -7.025792437124636392E-31 ) ) ;
#19031=ORIENTED_EDGE ( 'NONE', *, *, #9598, .T. ) ;
#19036=CARTESIAN_POINT ( 'NONE',  ( -3.414274948570314550, -9.020562075079396891E-14, -21.66938530120587814 ) ) ;
#19041=CARTESIAN_POINT ( 'NONE',  ( -3.414274948570314550, -0.5000000000000768274, -21.66938530120587814 ) ) ;
#19051=ORIENTED_EDGE ( 'NONE', *, *, #17691, .T. ) ;
#19054=CIRCLE ( 'NONE', #11906, 9.500000000000056843 ) ;
#19055=ORIENTED_EDGE ( 'NONE', *, *, #16274, .T. ) ;
#19066=CARTESIAN_POINT ( 'NONE',  ( -42.54314575050795355, 3.999999999999996447, -7.500000000000007105 ) ) ;
#19071=AXIS2_PLACEMENT_3D ( 'NONE', #16426, #21751, #5632 ) ;
#19072=CARTESIAN_POINT ( 'NONE',  ( -55.25320565519140104, -3.200000000000108979, 7.500000000000047962 ) ) ;
#19076=AXIS2_PLACEMENT_3D ( 'NONE', #2372, #6261, #18721 ) ;
#19085=AXIS2_PLACEMENT_3D ( 'NONE', #19802, #10853, #14617 ) ;
#19092=FACE_OUTER_BOUND ( 'NONE', #7004, .T. ) ;
#19094=VECTOR ( 'NONE', #17289, 1000.000000000000000 ) ;
#19096=AXIS2_PLACEMENT_3D ( 'NONE', #4656, #6549, #19119 ) ;
#19102=CARTESIAN_POINT ( 'NONE',  ( -50.65685424949281668, 0.5000000000000143219, 7.500000000000034639 ) ) ;
#19103=VERTEX_POINT ( 'NONE', #13027 ) ;
#19105=VERTEX_POINT ( 'NONE', #20320 ) ;
#19115=DIRECTION ( 'NONE',  ( -1.000000000000000000, 0.000000000000000000, 0.000000000000000000 ) ) ;
#19117=EDGE_CURVE ( 'NONE', #6327, #8147, #16653, .T. ) ;
#19119=DIRECTION ( 'NONE',  ( -1.000000000000000000, 6.938893903907186568E-15, 0.000000000000000000 ) ) ;
#19120=DIRECTION ( 'NONE',  ( 2.220446049250313081E-16, -1.000000000000000000, 7.025792437124636392E-31 ) ) ;
#19126=AXIS2_PLACEMENT_3D ( 'NONE', #2424, #9259, #2537 ) ;
#19132=CIRCLE ( 'NONE', #12392, 1.300000000000009592 ) ;
#19137=ORIENTED_EDGE ( 'NONE', *, *, #23210, .T. ) ;
#19140=EDGE_CURVE ( 'NONE', #18130, #11317, #17032, .T. ) ;
#19141=DIRECTION ( 'NONE',  ( -1.000000000000000000, 1.424116703980815236E-16, 2.931272055834072749E-32 ) ) ;
#19144=DIRECTION ( 'NONE',  ( 0.1556420233463076119, 0.000000000000000000, 0.9878135252003121813 ) ) ;
#19162=ORIENTED_EDGE ( 'NONE', *, *, #21177, .F. ) ;
#19165=EDGE_CURVE ( 'NONE', #19569, #5921, #18186, .T. ) ;
#19172=DIRECTION ( 'NONE',  ( -2.220446049250313081E-16, 1.000000000000000000, -7.025792437124636392E-31 ) ) ;
#19175=DIRECTION ( 'NONE',  ( 2.013525853228518840E-32, -6.902532920683810383E-31, 1.000000000000000000 ) ) ;
#19179=CARTESIAN_POINT ( 'NONE',  ( -90.63385214007837476, -2.700000000000084110, -7.926881151201908615 ) ) ;
#19184=DIRECTION ( 'NONE',  ( 1.550910762415566494E-16, 1.000000000000000000, -8.135128085091684243E-31 ) ) ;
#19208=LINE ( 'NONE', #6405, #3174 ) ;
#19218=ORIENTED_EDGE ( 'NONE', *, *, #336, .F. ) ;
#19233=FACE_OUTER_BOUND ( 'NONE', #22062, .T. ) ;
#19235=DIRECTION ( 'NONE',  ( 2.013525853228518840E-32, -6.902532920683810383E-31, 1.000000000000000000 ) ) ;
#19238=DIRECTION ( 'NONE',  ( 1.000000000000000000, -1.550910762415513985E-16, -3.012982189080959477E-32 ) ) ;
#19240=CARTESIAN_POINT ( 'NONE',  ( -90.55603112840530855, 4.857225732735059864E-14, -7.432974388601742533 ) ) ;
#19249=PRODUCT_DEFINITION_SHAPE ( 'NONE', 'NONE',  #11058 ) ;
#19252=DIRECTION ( 'NONE',  ( 0.2405376366294452728, 0.000000000000000000, -0.9706398123736327266 ) ) ;
#19253=CIRCLE ( 'NONE', #20513, 0.4999999999999994449 ) ;
#19258=VECTOR ( 'NONE', #20400, 1000.000000000000000 ) ;
#19262=AXIS2_PLACEMENT_3D ( 'NONE', #22333, #22213, #20810 ) ;
#19264=DIRECTION ( 'NONE',  ( 1.000000000000000000, 2.168404344970995063E-16, 6.201636426617045919E-15 ) ) ;
#19270=DIRECTION ( 'NONE',  ( 0.000000000000000000, 0.000000000000000000, -1.000000000000000000 ) ) ;
#19277=CIRCLE ( 'NONE', #1996, 0.5000000000000029976 ) ;
#19283=EDGE_CURVE ( 'NONE', #7855, #21664, #4883, .T. ) ;
#19289=CARTESIAN_POINT ( 'NONE',  ( -50.65685424949274562, 7.199999999999935341, -8.000000000000062172 ) ) ;
#19290=CARTESIAN_POINT ( 'NONE',  ( -43.10883117545719045, 4.565685424949256443, 7.500000000000007105 ) ) ;
#19295=AXIS2_PLACEMENT_3D ( 'NONE', #3595, #7473, #10873 ) ;
#19296=CARTESIAN_POINT ( 'NONE',  ( -6.746326818733273001, -2.700000000000056577, 27.22340457528592239 ) ) ;
#19298=DIRECTION ( 'NONE',  ( 1.000000000000000000, -1.734723475976793289E-15, -1.319263693449169988E-31 ) ) ;
#19301=EDGE_CURVE ( 'NONE', #13876, #1919, #6546, .T. ) ;
#19307=ORIENTED_EDGE ( 'NONE', *, *, #12230, .F. ) ;
#19308=ORIENTED_EDGE ( 'NONE', *, *, #6870, .F. ) ;
#19309=ADVANCED_FACE ( 'NONE', ( #14070 ), #10648, .F. ) ;
#19313=EDGE_CURVE ( 'NONE', #1694, #6466, #19721, .T. ) ;
#19315=AXIS2_PLACEMENT_3D ( 'NONE', #22750, #14036, #17439 ) ;
#19327=DIRECTION ( 'NONE',  ( -2.013525853228507892E-32, -6.902532920683810383E-31, 1.000000000000000000 ) ) ;
#19349=FACE_OUTER_BOUND ( 'NONE', #4674, .T. ) ;
#19350=ORIENTED_EDGE ( 'NONE', *, *, #4369, .F. ) ;
#19368=ADVANCED_FACE ( 'NONE', ( #16282 ), #3156, .T. ) ;
#19372=FACE_OUTER_BOUND ( 'NONE', #10593, .T. ) ;
#19374=DIRECTION ( 'NONE',  ( 1.000000000000000000, 0.000000000000000000, 0.000000000000000000 ) ) ;
#19378=DIRECTION ( 'NONE',  ( -2.013525853228507892E-32, -6.902532920683810383E-31, 1.000000000000000000 ) ) ;
#19382=LINE ( 'NONE', #22572, #22466 ) ;
#19386=CIRCLE ( 'NONE', #11483, 3.500000000000023981 ) ;
#19389=VERTEX_POINT ( 'NONE', #16163 ) ;
#19395=ORIENTED_EDGE ( 'NONE', *, *, #19117, .F. ) ;
#19402=AXIS2_PLACEMENT_3D ( 'NONE', #7248, #20060, #9352 ) ;
#19403=FACE_OUTER_BOUND ( 'NONE', #1382, .T. ) ;
#19420=ORIENTED_EDGE ( 'NONE', *, *, #9950, .T. ) ;
#19427=EDGE_CURVE ( 'NONE', #7622, #16517, #12640, .T. ) ;
#19429=LINE ( 'NONE', #1555, #23197 ) ;
#19439=CARTESIAN_POINT ( 'NONE',  ( -43.10883117545719045, 4.565685424949256443, 7.500000000000007105 ) ) ;
#19443=DIRECTION ( 'NONE',  ( -1.000000000000000000, 1.550910762415513985E-16, 3.012982189080959477E-32 ) ) ;
#19449=ORIENTED_EDGE ( 'NONE', *, *, #13056, .T. ) ;
#19466=DIRECTION ( 'NONE',  ( -0.1556420233463030045, -1.387778780781374185E-17, -0.9878135252003127365 ) ) ;
#19468=LINE ( 'NONE', #6763, #10881 ) ;
#19475=VECTOR ( 'NONE', #18962, 1000.000000000000000 ) ;
#19492=DIRECTION ( 'NONE',  ( -1.000000000000000000, 1.060108790874707909E-14, 0.000000000000000000 ) ) ;
#19494=AXIS2_PLACEMENT_3D ( 'NONE', #836, #13070, #4118 ) ;
#19496=DIRECTION ( 'NONE',  ( 1.000000000000000000, -1.389842848855773367E-62, 2.013525853228507892E-32 ) ) ;
#19507=LINE ( 'NONE', #12319, #6136 ) ;
#19519=EDGE_LOOP ( 'NONE', ( #10856, #5981, #12326, #17965 ) ) ;
#19520=AXIS2_PLACEMENT_3D ( 'NONE', #3186, #3302, #17516 ) ;
#19527=CARTESIAN_POINT ( 'NONE',  ( -89.70000000000054285, -0.5000000000000628386, 1.000000000000000888 ) ) ;
#19530=DIRECTION ( 'NONE',  ( -2.013525853228507892E-32, -6.902532920683810383E-31, 1.000000000000000000 ) ) ;
#19534=DIRECTION ( 'NONE',  ( -1.000000000000000000, 1.550910762415500426E-16, 0.000000000000000000 ) ) ;
#19539=ORIENTED_EDGE ( 'NONE', *, *, #10256, .F. ) ;
#19548=DIRECTION ( 'NONE',  ( -0.7453559924999295649, 0.000000000000000000, 0.6666666666666669627 ) ) ;
#19550=DIRECTION ( 'NONE',  ( -0.7071067811865505703, 0.7071067811865447972, -1.952833229202414720E-15 ) ) ;
#19556=CARTESIAN_POINT ( 'NONE',  ( -55.25320565519145788, 1.040834085586084257E-13, 10.00000000000009237 ) ) ;
#19569=VERTEX_POINT ( 'NONE', #4851 ) ;
#19571=ORIENTED_EDGE ( 'NONE', *, *, #8222, .T. ) ;
#19579=EDGE_CURVE ( 'NONE', #18130, #12501, #8443, .T. ) ;
#19583=CARTESIAN_POINT ( 'NONE',  ( -91.14322581977725690, -2.700000000000125855, 6.823838874241844543 ) ) ;
#19585=TOROIDAL_SURFACE ( 'NONE', #4549, 9.499999999999998224, 0.5000000000000000000 ) ;
#19592=ADVANCED_FACE ( 'NONE', ( #19092 ), #15325, .T. ) ;
#19595=ADVANCED_FACE ( 'NONE', ( #20640 ), #18984, .T. ) ;
#19598=ORIENTED_EDGE ( 'NONE', *, *, #16659, .F. ) ;
#19602=AXIS2_PLACEMENT_3D ( 'NONE', #17110, #1021, #15355 ) ;
#19604=EDGE_CURVE ( 'NONE', #11001, #5105, #2028, .T. ) ;
#19606=ORIENTED_EDGE ( 'NONE', *, *, #13816, .F. ) ;
#19608=ADVANCED_FACE ( 'NONE', ( #10729 ), #19912, .F. ) ;
#19609=CARTESIAN_POINT ( 'NONE',  ( -2.700000000000119194, 1.999999999999946265, -8.000000000000007105 ) ) ;
#19614=DIRECTION ( 'NONE',  ( -1.000000000000000000, 1.424116703980815236E-16, 2.931272055834072749E-32 ) ) ;
#19618=DIRECTION ( 'NONE',  ( -2.013525853228508439E-32, -6.779273404243028164E-31, 1.000000000000000000 ) ) ;
#19621=CARTESIAN_POINT ( 'NONE',  ( -42.54314575050793934, 5.299999999999998934, 7.500000000000062172 ) ) ;
#19623=CIRCLE ( 'NONE', #18491, 4.500000000000031974 ) ;
#19626=EDGE_LOOP ( 'NONE', ( #11111, #7486, #18670, #16999 ) ) ;
#19629=ADVANCED_FACE ( 'NONE', ( #3337 ), #18579, .T. ) ;
#19633=VECTOR ( 'NONE', #10291, 1000.000000000000000 ) ;
#19635=AXIS2_PLACEMENT_3D ( 'NONE', #19734, #1612, #7037 ) ;
#19645=LINE ( 'NONE', #7410, #20716 ) ;
#19650=DIRECTION ( 'NONE',  ( -2.220446049250313081E-16, 1.000000000000000000, -7.025792437124636392E-31 ) ) ;
#19659=EDGE_CURVE ( 'NONE', #1136, #10432, #14034, .T. ) ;
#19673=AXIS2_PLACEMENT_3D ( 'NONE', #5297, #19530, #1869 ) ;
#19674=FACE_OUTER_BOUND ( 'NONE', #8207, .T. ) ;
#19675=AXIS2_PLACEMENT_3D ( 'NONE', #19527, #10699, #14341 ) ;
#19676=CARTESIAN_POINT ( 'NONE',  ( -89.70000000000059970, 5.551115123125782702E-14, 1.000000000000000888 ) ) ;
#19689=CARTESIAN_POINT ( 'NONE',  ( -67.40537636629490237, -0.5000000000001045830, 12.70639812373640432 ) ) ;
#19697=VECTOR ( 'NONE', #6540, 1000.000000000000000 ) ;
#19702=EDGE_LOOP ( 'NONE', ( #14129, #17512, #4774, #5468 ) ) ;
#19703=ORIENTED_EDGE ( 'NONE', *, *, #4360, .F. ) ;
#19706=CARTESIAN_POINT ( 'NONE',  ( -50.65685424949275983, 7.200000000000018829, -8.000000000000007105 ) ) ;
#19717=LINE ( 'NONE', #19946, #11372 ) ;
#19720=LINE ( 'NONE', #6895, #9693 ) ;
#19721=LINE ( 'NONE', #12175, #10275 ) ;
#19727=FACE_OUTER_BOUND ( 'NONE', #22997, .T. ) ;
#19732=VECTOR ( 'NONE', #1552, 1000.000000000000000 ) ;
#19734=CARTESIAN_POINT ( 'NONE',  ( -55.25320565519140104, -3.200000000000108979, 10.00000000000007816 ) ) ;
#19736=CARTESIAN_POINT ( 'NONE',  ( -50.65685424949267457, -7.200000000000071232, -8.000000000000007105 ) ) ;
#19740=DIRECTION ( 'NONE',  ( -1.000000000000000000, -2.220446049250314067E-16, 5.825996348268307008E-33 ) ) ;
#19744=LINE ( 'NONE', #5275, #2824 ) ;
#19746=CIRCLE ( 'NONE', #218, 6.000000000000047073 ) ;
#19747=CARTESIAN_POINT ( 'NONE',  ( -47.47487373415324186, 4.018019484660552365, 8.000000000000062172 ) ) ;
#19748=DIRECTION ( 'NONE',  ( -1.000000000000000000, 1.626303258728244079E-16, 0.000000000000000000 ) ) ;
#19754=EDGE_LOOP ( 'NONE', ( #718, #23266, #805, #3304 ) ) ;
#19763=ORIENTED_EDGE ( 'NONE', *, *, #19659, .T. ) ;
#19769=DIRECTION ( 'NONE',  ( -1.550910762415566494E-16, -1.000000000000000000, 8.135128085091684243E-31 ) ) ;
#19780=VERTEX_POINT ( 'NONE', #2126 ) ;
#19784=ORIENTED_EDGE ( 'NONE', *, *, #18439, .T. ) ;
#19802=CARTESIAN_POINT ( 'NONE',  ( -47.47487373415321343, -4.018019484660608320, -7.500000000000007105 ) ) ;
#19805=EDGE_LOOP ( 'NONE', ( #20915, #6528, #2533, #18292 ) ) ;
#19808=ORIENTED_EDGE ( 'NONE', *, *, #10402, .T. ) ;
#19814=EDGE_LOOP ( 'NONE', ( #5704, #8607, #10623, #9505 ) ) ;
#19815=CARTESIAN_POINT ( 'NONE',  ( -50.65685424949274562, 7.200000000000025935, 17.71251237973613257 ) ) ;
#19826=CARTESIAN_POINT ( 'NONE',  ( -2.700000000000091216, -2.000000000000001776, -7.500000000000034639 ) ) ;
#19831=ORIENTED_EDGE ( 'NONE', *, *, #2034, .T. ) ;
#19838=VERTEX_POINT ( 'NONE', #8013 ) ;
#19841=ADVANCED_FACE ( 'NONE', ( #15641 ), #6600, .T. ) ;
#19847=CARTESIAN_POINT ( 'NONE',  ( -43.46238456605044576, -4.919238815542552601, 8.000000000000035527 ) ) ;
#19849=CARTESIAN_POINT ( 'NONE',  ( -55.25320565519150051, 0.5000000000000905942, 7.500000000000062172 ) ) ;
#19850=DIRECTION ( 'NONE',  ( 0.7071067811865495711, -0.7071067811865455743, -4.556821512286142627E-17 ) ) ;
#19863=ADVANCED_FACE ( 'NONE', ( #6717 ), #8359, .F. ) ;
#19867=DIRECTION ( 'NONE',  ( 0.9706398123736329486, -1.505375731439247187E-16, 0.2405376366294442458 ) ) ;
#19870=VERTEX_POINT ( 'NONE', #1314 ) ;
#19878=LINE ( 'NONE', #10472, #14196 ) ;
#19882=EDGE_CURVE ( 'NONE', #477, #19955, #7334, .T. ) ;
#19886=CARTESIAN_POINT ( 'NONE',  ( -50.65685424949280247, 1.387778780781445676E-14, 8.000000000000090594 ) ) ;
#19890=DIRECTION ( 'NONE',  ( 1.550910762415566494E-16, 1.000000000000000000, -8.135128085091684243E-31 ) ) ;
#19894=EDGE_CURVE ( 'NONE', #8929, #22821, #20723, .T. ) ;
#19901=ORIENTED_EDGE ( 'NONE', *, *, #17854, .F. ) ;
#19902=ORIENTED_EDGE ( 'NONE', *, *, #20442, .F. ) ;
#19911=DIRECTION ( 'NONE',  ( -1.000000000000000000, 1.550910762415566494E-16, -8.566929763922626680E-48 ) ) ;
#19912=CYLINDRICAL_SURFACE ( 'NONE', #4670, 2.800000000000017142 ) ;
#19916=APPLICATION_CONTEXT ( 'automotive_design' ) ;
#19919=DIRECTION ( 'NONE',  ( -2.013525853228518840E-32, 6.902532920683810383E-31, -1.000000000000000000 ) ) ;
#19922=CYLINDRICAL_SURFACE ( 'NONE', #20554, 0.5000000000000037748 ) ;
#19923=ORIENTED_EDGE ( 'NONE', *, *, #5106, .F. ) ;
#19928=ORIENTED_EDGE ( 'NONE', *, *, #1783, .T. ) ;
#19930=VERTEX_POINT ( 'NONE', #11994 ) ;
#19939=DIRECTION ( 'NONE',  ( 0.7071067811865268116, -0.7071067811865682229, -1.010793663541205907E-16 ) ) ;
#19940=CARTESIAN_POINT ( 'NONE',  ( -95.70000000000058549, -1.318389841742373392E-13, 1.000000000000014655 ) ) ;
#19943=DIRECTION ( 'NONE',  ( 0.7071067811865485719, -0.7071067811865464625, -1.010793663541191362E-16 ) ) ;
#19946=CARTESIAN_POINT ( 'NONE',  ( -66.55000000000046612, 6.188383139260622304E-14, -1.999999999999974021 ) ) ;
#19952=ORIENTED_EDGE ( 'NONE', *, *, #15288, .T. ) ;
#19953=ORIENTED_EDGE ( 'NONE', *, *, #10256, .T. ) ;
#19955=VERTEX_POINT ( 'NONE', #6961 ) ;
#19959=AXIS2_PLACEMENT_3D ( 'NONE', #2893, #10073, #6318 ) ;
#19969=CARTESIAN_POINT ( 'NONE',  ( -45.37157287525418781, 6.828427124746204058, -7.500000000000007105 ) ) ;
#19973=TOROIDAL_SURFACE ( 'NONE', #19602, 2.500000000000003997, 0.5000000000000000000 ) ;
#19978=DIRECTION ( 'NONE',  ( -1.000000000000000000, 1.389842848855773367E-62, -2.013525853228507892E-32 ) ) ;
#19991=CARTESIAN_POINT ( 'NONE',  ( -6.000000000000130562, 1.999999999999960032, -8.000000000000035527 ) ) ;
#19992=LINE ( 'NONE', #5655, #23217 ) ;
#19997=STYLED_ITEM ( 'NONE', ( #11567 ), #5304 ) ;
#19999=EDGE_CURVE ( 'NONE', #20601, #8098, #21974, .T. ) ;
#20005=EDGE_CURVE ( 'NONE', #18914, #11721, #3423, .T. ) ;
#20018=CYLINDRICAL_SURFACE ( 'NONE', #14173, 0.5000000000000000000 ) ;
#20019=EDGE_CURVE ( 'NONE', #4165, #13876, #12947, .T. ) ;
#20035=EDGE_CURVE ( 'NONE', #17272, #7855, #4691, .T. ) ;
#20041=ORIENTED_EDGE ( 'NONE', *, *, #12022, .T. ) ;
#20048=ORIENTED_EDGE ( 'NONE', *, *, #18652, .F. ) ;
#20054=DIRECTION ( 'NONE',  ( -1.298062744027682297E-32, 6.902532920683810383E-31, -1.000000000000000000 ) ) ;
#20055=DIRECTION ( 'NONE',  ( -2.220446049250313081E-16, 1.000000000000000000, -7.025792437124636392E-31 ) ) ;
#20060=DIRECTION ( 'NONE',  ( 0.9706398123736300620, 1.281898970984135951E-30, 0.2405376366294562085 ) ) ;
#20068=FACE_OUTER_BOUND ( 'NONE', #21248, .T. ) ;
#20074=EDGE_CURVE ( 'NONE', #3004, #1433, #18591, .T. ) ;
#20081=DIRECTION ( 'NONE',  ( 1.000000000000000000, -1.389842848855773367E-62, 2.013525853228507892E-32 ) ) ;
#20084=CARTESIAN_POINT ( 'NONE',  ( -61.45000000000039364, -3.200000000000081890, -2.000000000000002220 ) ) ;
#20091=EDGE_CURVE ( 'NONE', #2848, #6243, #17845, .T. ) ;
#20092=FACE_BOUND ( 'NONE', #5244, .T. ) ;
#20093=AXIS2_PLACEMENT_3D ( 'NONE', #5183, #5536, #17523 ) ;
#20098=ORIENTED_EDGE ( 'NONE', *, *, #21858, .F. ) ;
#20108=DIRECTION ( 'NONE',  ( -2.220446049250313081E-16, 1.000000000000000000, -7.025792437124636392E-31 ) ) ;
#20111=CARTESIAN_POINT ( 'NONE',  ( -90.55603112840530855, 2.700000000000056577, -7.432974388601742533 ) ) ;
#20123=EDGE_LOOP ( 'NONE', ( #7907, #2672 ) ) ;
#20126=DIRECTION ( 'NONE',  ( -1.000000000000000000, 1.445602896647327823E-16, 0.000000000000000000 ) ) ;
#20127=EDGE_CURVE ( 'NONE', #16517, #6243, #13342, .T. ) ;
#20130=AXIS2_PLACEMENT_3D ( 'NONE', #9894, #964, #15292 ) ;
#20142=DIRECTION ( 'NONE',  ( -1.000000000000000000, -1.479114197289387852E-30, 2.013525853228518840E-32 ) ) ;
#20143=CIRCLE ( 'NONE', #20538, 2.000000000000015543 ) ;
#20154=ORIENTED_EDGE ( 'NONE', *, *, #10947, .F. ) ;
#20162=EDGE_CURVE ( 'NONE', #13948, #12565, #9189, .T. ) ;
#20164=DIRECTION ( 'NONE',  ( 1.815210279346896549E-30, -6.902532920684321857E-31, 1.000000000000000000 ) ) ;
#20165=VECTOR ( 'NONE', #10889, 1000.000000000000000 ) ;
#20173=EDGE_CURVE ( 'NONE', #16292, #4603, #13171, .T. ) ;
#20190=VECTOR ( 'NONE', #22723, 1000.000000000000000 ) ;
#20192=AXIS2_PLACEMENT_3D ( 'NONE', #22129, #7551, #3896 ) ;
#20196=CIRCLE ( 'NONE', #7053, 2.000000000000015543 ) ;
#20199=EDGE_CURVE ( 'NONE', #18669, #19569, #15262, .T. ) ;
#20205=DIRECTION ( 'NONE',  ( 0.2405376366294550983, 0.000000000000000000, -0.9706398123736303951 ) ) ;
#20213=SHAPE_REPRESENTATION_RELATIONSHIP ( 'NONE' , 'NONE' ,  #20536, #15045 ) ;
#20218=VECTOR ( 'NONE', #8167, 1000.000000000000114 ) ;
#20221=ORIENTED_EDGE ( 'NONE', *, *, #3592, .F. ) ;
#20229=DIRECTION ( 'NONE',  ( -1.000000000000000000, -2.220446049250318011E-16, 0.000000000000000000 ) ) ;
#20239=LINE ( 'NONE', #7755, #6566 ) ;
#20246=CIRCLE ( 'NONE', #22494, 5.500000000000032863 ) ;
#20249=EDGE_LOOP ( 'NONE', ( #21611, #8720, #1124, #5228 ) ) ;
#20250=CARTESIAN_POINT ( 'NONE',  ( -95.70000000000069917, 2.775557561562891351E-14, 8.000000000000090594 ) ) ;
#20254=ORIENTED_EDGE ( 'NONE', *, *, #11233, .T. ) ;
#20257=DIRECTION ( 'NONE',  ( 0.7071067811865490160, 0.7071067811865460184, 1.565905175853767167E-16 ) ) ;
#20258=DIRECTION ( 'NONE',  ( 2.013525853228507892E-32, 6.902532920683810383E-31, -1.000000000000000000 ) ) ;
#20269=CARTESIAN_POINT ( 'NONE',  ( -55.05572809000125289, -0.5000000000001045830, -10.00000000000006395 ) ) ;
#20271=VERTEX_POINT ( 'NONE', #16909 ) ;
#20274=ORIENTED_EDGE ( 'NONE', *, *, #19117, .T. ) ;
#20280=EDGE_LOOP ( 'NONE', ( #19449, #7571, #63, #16200 ) ) ;
#20285=AXIS2_PLACEMENT_3D ( 'NONE', #5174, #14114, #10344 ) ;
#20286=DIRECTION ( 'NONE',  ( -1.393974221767077062E-14, -1.000000000000000000, 0.000000000000000000 ) ) ;
#20288=DIRECTION ( 'NONE',  ( -2.220446049250313081E-16, 1.000000000000000000, -7.025792437124636392E-31 ) ) ;
#20293=FILL_AREA_STYLE ('',( #14873 ) ) ;
#20301=ORIENTED_EDGE ( 'NONE', *, *, #1339, .F. ) ;
#20310=EDGE_LOOP ( 'NONE', ( #17302, #21472, #23091, #16398 ) ) ;
#20312=FACE_OUTER_BOUND ( 'NONE', #20421, .T. ) ;
#20317=EDGE_CURVE ( 'NONE', #11317, #10432, #8468, .T. ) ;
#20319=DIRECTION ( 'NONE',  ( 0.000000000000000000, 0.000000000000000000, 1.000000000000000000 ) ) ;
#20320=CARTESIAN_POINT ( 'NONE',  ( -6.000000000000074607, -4.800000000000026468, -7.500000000000034639 ) ) ;
#20322=PRESENTATION_STYLE_ASSIGNMENT (( #2434 ) ) ;
#20331=DIRECTION ( 'NONE',  ( 0.9878135252003128475, -1.532010627492774680E-16, -0.1556420233463030045 ) ) ;
#20333=ORIENTED_EDGE ( 'NONE', *, *, #12703, .F. ) ;
#20335=DIRECTION ( 'NONE',  ( -1.550910762415566494E-16, -1.000000000000000000, 8.135128085091684243E-31 ) ) ;
#20338=CARTESIAN_POINT ( 'NONE',  ( -64.00000000000045475, 3.200000000000057021, -1.999999999999974021 ) ) ;
#20339=CARTESIAN_POINT ( 'NONE',  ( -64.00000000000038369, -2.700000000000091216, -2.000000000000029310 ) ) ;
#20343=AXIS2_PLACEMENT_3D ( 'NONE', #7495, #5273, #21404 ) ;
#20345=FACE_OUTER_BOUND ( 'NONE', #16150, .T. ) ;
#20356=DIRECTION ( 'NONE',  ( 1.000000000000000000, 1.725633230170952464E-30, -1.831867990631496853E-15 ) ) ;
#20363=CARTESIAN_POINT ( 'NONE',  ( -42.54314575050793934, 3.999999999999996447, 7.500000000000062172 ) ) ;
#20371=DIRECTION ( 'NONE',  ( -2.013525853228507892E-32, -6.902532920683810383E-31, 1.000000000000000000 ) ) ;
#20385=EDGE_LOOP ( 'NONE', ( #13356, #14132, #4950, #1270 ) ) ;
#20395=DIRECTION ( 'NONE',  ( 0.000000000000000000, 0.000000000000000000, 1.000000000000000000 ) ) ;
#20398=CARTESIAN_POINT ( 'NONE',  ( -89.70000000000064233, 4.857225732735059864E-14, -2.000000000000001776 ) ) ;
#20400=DIRECTION ( 'NONE',  ( 2.013525853228507892E-32, 6.902532920683810383E-31, -1.000000000000000000 ) ) ;
#20406=DIRECTION ( 'NONE',  ( -2.220446049250313081E-16, 1.000000000000000000, -7.025792437124636392E-31 ) ) ;
#20421=EDGE_LOOP ( 'NONE', ( #1631, #15273, #14483, #7150 ) ) ;
#20427=CARTESIAN_POINT ( 'NONE',  ( -55.25320565519152893, 0.5000000000000905942, 8.000000000000035527 ) ) ;
#20429=AXIS2_PLACEMENT_3D ( 'NONE', #2574, #22573, #13637 ) ;
#20438=LINE ( 'NONE', #15122, #6355 ) ;
#20442=EDGE_CURVE ( 'NONE', #13984, #10886, #19744, .T. ) ;
#20468=EDGE_CURVE ( 'NONE', #22523, #8174, #1733, .T. ) ;
#20475=EDGE_CURVE ( 'NONE', #16835, #21928, #13728, .T. ) ;
#20486=LINE ( 'NONE', #17161, #17862 ) ;
#20495=EDGE_CURVE ( 'NONE', #1910, #7626, #14896, .T. ) ;
#20498=CARTESIAN_POINT ( 'NONE',  ( -6.000000000000130562, 7.499999999999958256, -8.000000000000035527 ) ) ;
#20507=ORIENTED_EDGE ( 'NONE', *, *, #9671, .F. ) ;
#20513=AXIS2_PLACEMENT_3D ( 'NONE', #10354, #22959, #10133 ) ;
#20522=DIRECTION ( 'NONE',  ( 0.000000000000000000, 0.000000000000000000, -1.000000000000000000 ) ) ;
#20532=DIRECTION ( 'NONE',  ( 1.000000000000000000, -1.424116703980815236E-16, -2.931272055834072749E-32 ) ) ;
#20536=SHAPE_REPRESENTATION ( 'Hold Down Arm', ( #22115 ), #12708 ) ;
#20537=VERTEX_POINT ( 'NONE', #3726 ) ;
#20538=AXIS2_PLACEMENT_3D ( 'NONE', #5171, #12333, #3414 ) ;
#20554=AXIS2_PLACEMENT_3D ( 'NONE', #9092, #1905, #4131 ) ;
#20561=VECTOR ( 'NONE', #21048, 1000.000000000000000 ) ;
#20567=FACE_BOUND ( 'NONE', #5462, .T. ) ;
#20569=VERTEX_POINT ( 'NONE', #10896 ) ;
#20574=CARTESIAN_POINT ( 'NONE',  ( -65.47859922179029013, -6.938893903907228378E-14, -11.38422848940298593 ) ) ;
#20576=AXIS2_PLACEMENT_3D ( 'NONE', #460, #14919, #9515 ) ;
#20583=CARTESIAN_POINT ( 'NONE',  ( -95.20000000000065654, 6.938893903907228378E-15, 8.000000000000076383 ) ) ;
#20584=CARTESIAN_POINT ( 'NONE',  ( -6.000000000000047073, -7.500000000000003553, 8.000000000000090594 ) ) ;
#20585=AXIS2_PLACEMENT_3D ( 'NONE', #10159, #9933, #2636 ) ;
#20588=CIRCLE ( 'NONE', #18329, 10.00000000000006395 ) ;
#20591=EDGE_CURVE ( 'NONE', #14824, #19870, #15807, .T. ) ;
#20594=VECTOR ( 'NONE', #14478, 1000.000000000000000 ) ;
#20595=EDGE_LOOP ( 'NONE', ( #15937, #14312, #19606, #5723 ) ) ;
#20601=VERTEX_POINT ( 'NONE', #11832 ) ;
#20602=DIRECTION ( 'NONE',  ( -0.9878135252003120703, -1.380506584136762427E-30, 0.1556420233463082226 ) ) ;
#20610=AXIS2_PLACEMENT_3D ( 'NONE', #23161, #19378, #21513 ) ;
#20632=ORIENTED_EDGE ( 'NONE', *, *, #8889, .T. ) ;
#20636=AXIS2_PLACEMENT_3D ( 'NONE', #10074, #20675, #3136 ) ;
#20637=DIRECTION ( 'NONE',  ( 1.000000000000000000, 2.220446049250314067E-16, -5.825996348268307008E-33 ) ) ;
#20638=DIRECTION ( 'NONE',  ( -1.000000000000000000, 1.389842848855773367E-62, -2.013525853228507892E-32 ) ) ;
#20640=FACE_OUTER_BOUND ( 'NONE', #23178, .T. ) ;
#20642=CARTESIAN_POINT ( 'NONE',  ( -45.56568542494959928, -2.108831175456959972, -8.000000000000035527 ) ) ;
#20656=EDGE_CURVE ( 'NONE', #1880, #3212, #1190, .T. ) ;
#20665=DIRECTION ( 'NONE',  ( -0.8122328620674128530, 0.000000000000000000, -0.5833333333333344806 ) ) ;
#20669=DIRECTION ( 'NONE',  ( 1.000000000000000000, 0.000000000000000000, 0.000000000000000000 ) ) ;
#20675=DIRECTION ( 'NONE',  ( 2.220446049250314067E-16, -1.000000000000000000, 7.025792437124636392E-31 ) ) ;
#20676=AXIS2_PLACEMENT_3D ( 'NONE', #12755, #20054, #5933 ) ;
#20693=LINE ( 'NONE', #15148, #14343 ) ;
#20696=FACE_OUTER_BOUND ( 'NONE', #400, .T. ) ;
#20698=EDGE_CURVE ( 'NONE', #11721, #15489, #14331, .T. ) ;
#20706=ORIENTED_EDGE ( 'NONE', *, *, #883, .F. ) ;
#20716=VECTOR ( 'NONE', #14580, 1000.000000000000000 ) ;
#20718=CARTESIAN_POINT ( 'NONE',  ( -50.65685424949274562, 3.200000000000022382, -8.000000000000062172 ) ) ;
#20719=LINE ( 'NONE', #2834, #9428 ) ;
#20721=ADVANCED_FACE ( 'NONE', ( #15812 ), #6894, .T. ) ;
#20723=LINE ( 'NONE', #12106, #15189 ) ;
#20724=CARTESIAN_POINT ( 'NONE',  ( -42.54314575050782565, -7.500000000000038192, -8.000000000000007105 ) ) ;
#20726=DIRECTION ( 'NONE',  ( 1.734723475976805517E-15, 1.000000000000000000, 0.000000000000000000 ) ) ;
#20728=EDGE_CURVE ( 'NONE', #4887, #9452, #10921, .T. ) ;
#20737=AXIS2_PLACEMENT_3D ( 'NONE', #5760, #19550, #21092 ) ;
#20751=VECTOR ( 'NONE', #7585, 1000.000000000000000 ) ;
#20755=DIRECTION ( 'NONE',  ( 1.000000000000000000, 0.000000000000000000, 0.000000000000000000 ) ) ;
#20764=FACE_OUTER_BOUND ( 'NONE', #18466, .T. ) ;
#20771=EDGE_LOOP ( 'NONE', ( #4754, #18362, #10624, #13883 ) ) ;
#20806=EDGE_LOOP ( 'NONE', ( #5083, #16372, #425, #7736 ) ) ;
#20810=DIRECTION ( 'NONE',  ( 0.000000000000000000, 7.806255641895571971E-15, 1.000000000000000000 ) ) ;
#20813=ORIENTED_EDGE ( 'NONE', *, *, #3221, .F. ) ;
#20814=VECTOR ( 'NONE', #13395, 1000.000000000000000 ) ;
#20815=CARTESIAN_POINT ( 'NONE',  ( -43.10883117545714782, -5.300000000000020250, 7.500000000000062172 ) ) ;
#20828=CARTESIAN_POINT ( 'NONE',  ( -64.00000000000045475, -0.5000000000000628386, -2.000000000000001776 ) ) ;
#20831=DIRECTION ( 'NONE',  ( 1.000000000000000000, -1.389842848855773367E-62, 2.013525853228507892E-32 ) ) ;
#20833=AXIS2_PLACEMENT_3D ( 'NONE', #10535, #17592, #14304 ) ;
#20840=ORIENTED_EDGE ( 'NONE', *, *, #4318, .T. ) ;
#20845=ORIENTED_EDGE ( 'NONE', *, *, #11027, .F. ) ;
#20847=LINE ( 'NONE', #1309, #18371 ) ;
#20851=DIRECTION ( 'NONE',  ( -1.000000000000000000, 0.000000000000000000, 0.000000000000000000 ) ) ;
#20864=ORIENTED_EDGE ( 'NONE', *, *, #17919, .F. ) ;
#20867=CARTESIAN_POINT ( 'NONE',  ( -65.00000000000046896, -6.245004513516505540E-14, 3.000000000000030198 ) ) ;
#20876=CARTESIAN_POINT ( 'NONE',  ( -55.05572809000130974, 0.5000000000000143219, -8.000000000000035527 ) ) ;
#20885=EDGE_CURVE ( 'NONE', #10125, #19105, #11160, .T. ) ;
#20888=ORIENTED_EDGE ( 'NONE', *, *, #4784, .T. ) ;
#20908=EDGE_CURVE ( 'NONE', #14335, #15165, #8255, .T. ) ;
#20915=ORIENTED_EDGE ( 'NONE', *, *, #2601, .T. ) ;
#20922=EDGE_CURVE ( 'NONE', #23066, #19389, #19054, .T. ) ;
#20926=LINE ( 'NONE', #15377, #1224 ) ;
#20938=EDGE_LOOP ( 'NONE', ( #12978, #5307 ) ) ;
#20944=CARTESIAN_POINT ( 'NONE',  ( -89.70000000000057128, -9.020562075079396891E-14, -2.000000000000001776 ) ) ;
#20946=DIRECTION ( 'NONE',  ( -1.000000000000000000, -2.220446049250301001E-16, 0.000000000000000000 ) ) ;
#20949=ORIENTED_EDGE ( 'NONE', *, *, #20173, .F. ) ;
#20967=EDGE_LOOP ( 'NONE', ( #14503, #8292, #16496, #11540 ) ) ;
#20972=ORIENTED_EDGE ( 'NONE', *, *, #12659, .F. ) ;
#20978=DIRECTION ( 'NONE',  ( -1.000000000000000000, 1.389842848855773367E-62, -2.013525853228507892E-32 ) ) ;
#20982=CARTESIAN_POINT ( 'NONE',  ( -6.000000000000116351, 1.999999999999960032, -7.500000000000062172 ) ) ;
#20986=CARTESIAN_POINT ( 'NONE',  ( -65.00000000000046896, -0.5000000000000628386, 3.000000000000030198 ) ) ;
#21005=ORIENTED_EDGE ( 'NONE', *, *, #11510, .T. ) ;
#21006=DIRECTION ( 'NONE',  ( -1.550910762415566494E-16, -1.000000000000000000, 8.135128085091684243E-31 ) ) ;
#21010=CYLINDRICAL_SURFACE ( 'NONE', #9327, 7.200000000000022382 ) ;
#21013=EDGE_CURVE ( 'NONE', #2139, #8929, #22820, .T. ) ;
#21016=AXIS2_PLACEMENT_3D ( 'NONE', #10657, #17841, #1717 ) ;
#21018=DIRECTION ( 'NONE',  ( 0.9878135252003127365, -1.532010627492774434E-16, -0.1556420233463029767 ) ) ;
#21019=CARTESIAN_POINT ( 'NONE',  ( -56.91911807125104872, -1.040834085586084257E-13, -8.333333333333413862 ) ) ;
#21028=ORIENTED_EDGE ( 'NONE', *, *, #3704, .T. ) ;
#21033=DIRECTION ( 'NONE',  ( -1.000000000000000000, 1.389842848855773151E-62, -2.013525853228507618E-32 ) ) ;
#21037=CARTESIAN_POINT ( 'NONE',  ( -55.25320565519145788, -0.5000000000000281997, 10.00000000000009237 ) ) ;
#21040=EDGE_CURVE ( 'NONE', #9098, #21240, #17937, .T. ) ;
#21045=CARTESIAN_POINT ( 'NONE',  ( -89.70000000000059970, 2.700000000000056577, 1.000000000000000888 ) ) ;
#21048=DIRECTION ( 'NONE',  ( -1.550910762415566494E-16, -1.000000000000000000, 8.135128085091684243E-31 ) ) ;
#21051=EDGE_CURVE ( 'NONE', #6614, #20569, #15279, .T. ) ;
#21052=CYLINDRICAL_SURFACE ( 'NONE', #15324, 0.5000000000000029976 ) ;
#21057=ORIENTED_EDGE ( 'NONE', *, *, #14869, .T. ) ;
#21061=CARTESIAN_POINT ( 'NONE',  ( -61.45000000000046469, -7.672331518739548870E-14, -2.000000000000002220 ) ) ;
#21063=CARTESIAN_POINT ( 'NONE',  ( -3.200000000000036149, -7.500000000000027534, -7.500000000000007105 ) ) ;
#21067=FACE_OUTER_BOUND ( 'NONE', #20771, .T. ) ;
#21070=DIRECTION ( 'NONE',  ( -2.013525853228518840E-32, 6.902532920683810383E-31, -1.000000000000000000 ) ) ;
#21081=ORIENTED_EDGE ( 'NONE', *, *, #2920, .F. ) ;
#21083=EDGE_LOOP ( 'NONE', ( #748, #14765, #2944, #17925 ) ) ;
#21092=DIRECTION ( 'NONE',  ( -0.7071067811865457964, -0.7071067811865492381, 0.000000000000000000 ) ) ;
#21102=CYLINDRICAL_SURFACE ( 'NONE', #8905, 2.000000000000015543 ) ;
#21105=AXIS2_PLACEMENT_3D ( 'NONE', #228, #18339, #3330 ) ;
#21114=EDGE_LOOP ( 'NONE', ( #19420, #8341, #9914, #14678 ) ) ;
#21118=VERTEX_POINT ( 'NONE', #11394 ) ;
#21124=DIRECTION ( 'NONE',  ( -1.000000000000000000, 1.517883041479696593E-16, -5.334274688628647894E-15 ) ) ;
#21125=DIRECTION ( 'NONE',  ( -1.550910762415566494E-16, -1.000000000000000000, 8.135128085091684243E-31 ) ) ;
#21126=CARTESIAN_POINT ( 'NONE',  ( -6.000000000000088818, -2.000000000000043521, -7.500000000000007105 ) ) ;
#21138=DIRECTION ( 'NONE',  ( 2.220446049250313081E-16, -1.000000000000000000, 7.025792437124636392E-31 ) ) ;
#21143=AXIS2_PLACEMENT_3D ( 'NONE', #11009, #18540, #3953 ) ;
#21149=ADVANCED_FACE ( 'NONE', ( #2819 ), #997, .T. ) ;
#21151=DIRECTION ( 'NONE',  ( 2.013525853228507892E-32, 6.902532920683810383E-31, -1.000000000000000000 ) ) ;
#21157=CIRCLE ( 'NONE', #10995, 0.5000000000000029976 ) ;
#21158=DIRECTION ( 'NONE',  ( -2.220446049250313081E-16, 1.000000000000000000, -7.025792437124636392E-31 ) ) ;
#21159=DIRECTION ( 'NONE',  ( -1.387778780781437314E-14, 0.000000000000000000, 1.000000000000000000 ) ) ;
#21168=DIRECTION ( 'NONE',  ( -1.550910762415566494E-16, -1.000000000000000000, 8.135128085091684243E-31 ) ) ;
#21171=EDGE_CURVE ( 'NONE', #15244, #4366, #19386, .T. ) ;
#21177=EDGE_CURVE ( 'NONE', #1883, #4862, #17886, .T. ) ;
#21179=CIRCLE ( 'NONE', #893, 9.500000000000063949 ) ;
#21181=ORIENTED_EDGE ( 'NONE', *, *, #1645, .T. ) ;
#21185=LINE ( 'NONE', #12213, #13359 ) ;
#21188=ORIENTED_EDGE ( 'NONE', *, *, #18875, .T. ) ;
#21189=DIRECTION ( 'NONE',  ( 0.9706398123736329486, 2.155253336630096462E-16, 0.2405376366294442458 ) ) ;
#21194=DIRECTION ( 'NONE',  ( 1.000000000000000000, 2.168404344970991858E-16, 0.000000000000000000 ) ) ;
#21197=CARTESIAN_POINT ( 'NONE',  ( -3.200000000000049916, 1.999999999999911626, 7.999999999999979572 ) ) ;
#21198=AXIS2_PLACEMENT_3D ( 'NONE', #7635, #13045, #9629 ) ;
#21201=AXIS2_PLACEMENT_3D ( 'NONE', #20815, #4681, #2915 ) ;
#21202=FACE_BOUND ( 'NONE', #3655, .T. ) ;
#21203=EDGE_CURVE ( 'NONE', #14933, #22149, #17148, .T. ) ;
#21206=EDGE_CURVE ( 'NONE', #21952, #1880, #10364, .T. ) ;
#21208=VERTEX_POINT ( 'NONE', #20584 ) ;
#21210=ORIENTED_EDGE ( 'NONE', *, *, #8635, .T. ) ;
#21212=VERTEX_POINT ( 'NONE', #10332 ) ;
#21213=ORIENTED_EDGE ( 'NONE', *, *, #1693, .F. ) ;
#21219=CARTESIAN_POINT ( 'NONE',  ( -56.91911807125113398, 2.700000000000056577, -8.333333333333387216 ) ) ;
#21228=DIRECTION ( 'NONE',  ( -1.000000000000000000, -2.220446049250301001E-16, 0.000000000000000000 ) ) ;
#21232=VECTOR ( 'NONE', #14809, 1000.000000000000000 ) ;
#21240=VERTEX_POINT ( 'NONE', #11975 ) ;
#21241=ORIENTED_EDGE ( 'NONE', *, *, #20162, .F. ) ;
#21248=EDGE_LOOP ( 'NONE', ( #929, #13239, #4643, #5694 ) ) ;
#21260=DIRECTION ( 'NONE',  ( -0.7071067811865505703, 0.7071067811865444641, 1.010793663541190129E-16 ) ) ;
#21262=ORIENTED_EDGE ( 'NONE', *, *, #7216, .F. ) ;
#21269=ORIENTED_EDGE ( 'NONE', *, *, #12121, .T. ) ;
#21272=DIRECTION ( 'NONE',  ( -2.710505431213761578E-16, 1.000000000000000000, -7.518830502887770522E-31 ) ) ;
#21273=DIRECTION ( 'NONE',  ( -0.9706398123736329486, -2.155253336630096462E-16, -0.2405376366294442458 ) ) ;
#21274=CARTESIAN_POINT ( 'NONE',  ( -89.70000000000064233, 0.5000000000000490719, -2.000000000000001776 ) ) ;
#21283=EDGE_CURVE ( 'NONE', #2097, #22821, #18814, .T. ) ;
#21292=VECTOR ( 'NONE', #96, 1000.000000000000000 ) ;
#21298=VECTOR ( 'NONE', #15474, 1000.000000000000000 ) ;
#21301=CIRCLE ( 'NONE', #14157, 0.5000000000000019984 ) ;
#21304=AXIS2_PLACEMENT_3D ( 'NONE', #18486, #7446, #16481 ) ;
#21311=FACE_OUTER_BOUND ( 'NONE', #14080, .T. ) ;
#21315=DIRECTION ( 'NONE',  ( -1.000000000000000000, -2.220446049250301001E-16, 0.000000000000000000 ) ) ;
#21317=AXIS2_PLACEMENT_3D ( 'NONE', #6148, #2488, #15063 ) ;
#21332=DIRECTION ( 'NONE',  ( 1.000000000000000000, 1.479114197289387852E-30, -2.013525853228518840E-32 ) ) ;
#21345=CARTESIAN_POINT ( 'NONE',  ( -56.54644007500103697, -2.700000000000084110, -8.666666666666710483 ) ) ;
#21346=AXIS2_PLACEMENT_3D ( 'NONE', #2869, #15670, #13805 ) ;
#21349=DIRECTION ( 'NONE',  ( -1.000000000000000000, 2.168404344970992105E-16, 3.469446951953587368E-15 ) ) ;
#21361=ORIENTED_EDGE ( 'NONE', *, *, #11390, .F. ) ;
#21364=ORIENTED_EDGE ( 'NONE', *, *, #12267, .F. ) ;
#21366=AXIS2_PLACEMENT_3D ( 'NONE', #10237, #8137, #2842 ) ;
#21382=EDGE_LOOP ( 'NONE', ( #21810, #22638, #7300, #4923 ) ) ;
#21390=ADVANCED_FACE ( 'NONE', ( #7730, #20092, #680 ), #15013, .F. ) ;
#21395=VECTOR ( 'NONE', #4822, 1000.000000000000227 ) ;
#21404=DIRECTION ( 'NONE',  ( -1.000000000000000000, 0.000000000000000000, 0.000000000000000000 ) ) ;
#21422=DIRECTION ( 'NONE',  ( 0.000000000000000000, 0.000000000000000000, 1.000000000000000000 ) ) ;
#21427=EDGE_LOOP ( 'NONE', ( #13618, #16596, #15571, #15219 ) ) ;
#21429=CARTESIAN_POINT ( 'NONE',  ( -50.65685424949263904, -7.200000000000071232, -7.500000000000034639 ) ) ;
#21430=DIRECTION ( 'NONE',  ( 1.392757777031969319E-14, 1.000000000000000000, -5.941108692445745160E-30 ) ) ;
#21443=ORIENTED_EDGE ( 'NONE', *, *, #1321, .T. ) ;
#21457=DIRECTION ( 'NONE',  ( 1.000000000000000000, 0.000000000000000000, 0.000000000000000000 ) ) ;
#21472=ORIENTED_EDGE ( 'NONE', *, *, #13820, .T. ) ;
#21479=CARTESIAN_POINT ( 'NONE',  ( -43.46238456605044576, 4.919238815542508192, -7.500000000000034639 ) ) ;
#21482=EDGE_CURVE ( 'NONE', #4281, #1910, #9733, .T. ) ;
#21489=CARTESIAN_POINT ( 'NONE',  ( -65.00000000000052580, 2.700000000000063238, 3.000000000000002665 ) ) ;
#21490=DIRECTION ( 'NONE',  ( 1.000000000000000000, 1.479114197289388027E-30, -2.013525853228518840E-32 ) ) ;
#21496=DIRECTION ( 'NONE',  ( -0.8122328620674111876, 0.000000000000000000, -0.5833333333333368120 ) ) ;
#21499=EDGE_CURVE ( 'NONE', #3480, #10125, #8437, .T. ) ;
#21510=DIRECTION ( 'NONE',  ( -1.107262168541282614E-16, 1.107262168541365321E-16, -1.000000000000000000 ) ) ;
#21513=DIRECTION ( 'NONE',  ( 1.000000000000000000, 0.000000000000000000, 0.000000000000000000 ) ) ;
#21515=FACE_OUTER_BOUND ( 'NONE', #15213, .T. ) ;
#21517=DIRECTION ( 'NONE',  ( 2.013525853228507892E-32, 6.902532920683810383E-31, -1.000000000000000000 ) ) ;
#21518=AXIS2_PLACEMENT_3D ( 'NONE', #22100, #6338, #7864 ) ;
#21519=DIRECTION ( 'NONE',  ( -1.550910762415566494E-16, -1.000000000000000000, 8.135128085091684243E-31 ) ) ;
#21523=FACE_OUTER_BOUND ( 'NONE', #1603, .T. ) ;
#21525=ORIENTED_EDGE ( 'NONE', *, *, #14288, .T. ) ;
#21532=AXIS2_PLACEMENT_3D ( 'NONE', #3719, #10888, #18082 ) ;
#21536=TOROIDAL_SURFACE ( 'NONE', #14381, 4.500000000000002665, 0.5000000000000000000 ) ;
#21541=FACE_OUTER_BOUND ( 'NONE', #14907, .T. ) ;
#21542=EDGE_CURVE ( 'NONE', #19955, #18025, #15361, .T. ) ;
#21550=AXIS2_PLACEMENT_3D ( 'NONE', #22836, #6715, #10129 ) ;
#21551=AXIS2_PLACEMENT_3D ( 'NONE', #6193, #13364, #22889 ) ;
#21567=CYLINDRICAL_SURFACE ( 'NONE', #13177, 0.5000000000000004441 ) ;
#21584=CIRCLE ( 'NONE', #170, 0.5000000000000029976 ) ;
#21587=VECTOR ( 'NONE', #19006, 1000.000000000000114 ) ;
#21590=EDGE_LOOP ( 'NONE', ( #21758, #20632, #6436, #17423 ) ) ;
#21591=ORIENTED_EDGE ( 'NONE', *, *, #3625, .T. ) ;
#21604=EDGE_CURVE ( 'NONE', #15576, #9575, #17514, .T. ) ;
#21611=ORIENTED_EDGE ( 'NONE', *, *, #13106, .T. ) ;
#21617=ORIENTED_EDGE ( 'NONE', *, *, #21894, .T. ) ;
#21626=CARTESIAN_POINT ( 'NONE',  ( -6.000000000000074607, -4.800000000000026468, -7.500000000000034639 ) ) ;
#21630=ADVANCED_FACE ( 'NONE', ( #3479 ), #1595, .T. ) ;
#21644=VERTEX_POINT ( 'NONE', #21019 ) ;
#21645=DIRECTION ( 'NONE',  ( 2.013525853228507892E-32, 6.902532920683810383E-31, -1.000000000000000000 ) ) ;
#21653=DIRECTION ( 'NONE',  ( 0.000000000000000000, -1.000000000000000000, 0.000000000000000000 ) ) ;
#21660=DIRECTION ( 'NONE',  ( 1.000000000000000000, 2.168404344970995063E-16, 0.000000000000000000 ) ) ;
#21661=CARTESIAN_POINT ( 'NONE',  ( -55.25320565519145788, -4.163336342344337027E-14, 10.00000000000009237 ) ) ;
#21662=CARTESIAN_POINT ( 'NONE',  ( -89.70000000000064233, 5.551115123125782702E-14, -2.000000000000001776 ) ) ;
#21664=VERTEX_POINT ( 'NONE', #16049 ) ;
#21668=ORIENTED_EDGE ( 'NONE', *, *, #18570, .F. ) ;
#21704=FACE_OUTER_BOUND ( 'NONE', #22500, .T. ) ;
#21706=DIRECTION ( 'NONE',  ( -1.000000000000000000, -2.220446049250313081E-16, 0.000000000000000000 ) ) ;
#21717=CARTESIAN_POINT ( 'NONE',  ( -6.000000000000088818, -2.000000000000043521, 7.500000000000076383 ) ) ;
#21719=EDGE_LOOP ( 'NONE', ( #13503, #18078, #16254, #5786 ) ) ;
#21722=VERTEX_POINT ( 'NONE', #23141 ) ;
#21723=EDGE_LOOP ( 'NONE', ( #18532, #17213, #22412, #1402 ) ) ;
#21725=VERTEX_POINT ( 'NONE', #10991 ) ;
#21727=ORIENTED_EDGE ( 'NONE', *, *, #5798, .F. ) ;
#21735=CARTESIAN_POINT ( 'NONE',  ( -43.46238456605044576, 4.919238815542528620, 7.500000000000034639 ) ) ;
#21738=CARTESIAN_POINT ( 'NONE',  ( -89.70000000000057128, -9.020562075079396891E-14, -2.000000000000001776 ) ) ;
#21751=DIRECTION ( 'NONE',  ( 2.220446049250313081E-16, -1.000000000000000000, 7.025792437124636392E-31 ) ) ;
#21755=EDGE_CURVE ( 'NONE', #1743, #22996, #2170, .T. ) ;
#21756=AXIS2_PLACEMENT_3D ( 'NONE', #17913, #9079, #5324 ) ;
#21757=FACE_OUTER_BOUND ( 'NONE', #4141, .T. ) ;
#21758=ORIENTED_EDGE ( 'NONE', *, *, #1959, .F. ) ;
#21760=DIRECTION ( 'NONE',  ( -1.000000000000000000, 1.550910762415513985E-16, 3.012982189080959477E-32 ) ) ;
#21770=CARTESIAN_POINT ( 'NONE',  ( -6.000000000000130562, 1.999999999999960032, -8.000000000000035527 ) ) ;
#21791=CARTESIAN_POINT ( 'NONE',  ( -43.10883117545713361, -4.565685424949242233, 8.000000000000035527 ) ) ;
#21792=ADVANCED_FACE ( 'NONE', ( #18519 ), #13030, .T. ) ;
#21797=CARTESIAN_POINT ( 'NONE',  ( -45.91923881554284037, 2.462384566050156209, 8.000000000000076383 ) ) ;
#21802=VERTEX_POINT ( 'NONE', #15537 ) ;
#21810=ORIENTED_EDGE ( 'NONE', *, *, #557, .F. ) ;
#21811=ORIENTED_EDGE ( 'NONE', *, *, #1770, .F. ) ;
#21813=EDGE_LOOP ( 'NONE', ( #3458, #1383, #19539, #19218 ) ) ;
#21814=AXIS2_PLACEMENT_3D ( 'NONE', #7105, #4849, #20978 ) ;
#21819=DIRECTION ( 'NONE',  ( -1.000000000000000000, 2.785515554063903297E-14, 1.815210279346915817E-30 ) ) ;
#21826=DIRECTION ( 'NONE',  ( 1.331202777560457422E-30, 1.000000000000000000, -7.395570986446985676E-31 ) ) ;
#21837=ORIENTED_EDGE ( 'NONE', *, *, #8635, .F. ) ;
#21838=ORIENTED_EDGE ( 'NONE', *, *, #3507, .T. ) ;
#21849=CARTESIAN_POINT ( 'NONE',  ( -42.54314575050793934, 3.999999999999996447, 7.500000000000062172 ) ) ;
#21851=FACE_OUTER_BOUND ( 'NONE', #14968, .T. ) ;
#21855=DIRECTION ( 'NONE',  ( 2.013525853228518840E-32, -6.902532920683810383E-31, 1.000000000000000000 ) ) ;
#21858=EDGE_CURVE ( 'NONE', #7622, #8200, #5889, .T. ) ;
#21866=CARTESIAN_POINT ( 'NONE',  ( -89.70000000000064233, 3.200000000000057021, -2.000000000000001776 ) ) ;
#21870=CARTESIAN_POINT ( 'NONE',  ( -91.02295700146262902, 3.200000000000015277, 6.338518968055040226 ) ) ;
#21872=DIRECTION ( 'NONE',  ( -1.000000000000000000, -1.700709290173333260E-16, 0.000000000000000000 ) ) ;
#21876=DIRECTION ( 'NONE',  ( 1.000000000000000000, 1.600676661924044152E-14, 0.000000000000000000 ) ) ;
#21877=DIRECTION ( 'NONE',  ( 1.734723475976805517E-15, -1.000000000000000000, 0.000000000000000000 ) ) ;
#21878=LINE ( 'NONE', #14692, #21925 ) ;
#21879=CARTESIAN_POINT ( 'NONE',  ( -95.20000000000065654, -0.5000000000000975886, -2.000000000000001776 ) ) ;
#21882=EDGE_CURVE ( 'NONE', #21725, #6467, #22404, .T. ) ;
#21884=CIRCLE ( 'NONE', #15494, 5.500000000000032863 ) ;
#21886=AXIS2_PLACEMENT_3D ( 'NONE', #8561, #15724, #19374 ) ;
#21891=VERTEX_POINT ( 'NONE', #18869 ) ;
#21893=DIRECTION ( 'NONE',  ( -1.000000000000000000, -1.479114197289388027E-30, -2.013525853228507892E-32 ) ) ;
#21894=EDGE_CURVE ( 'NONE', #9575, #9299, #22287, .T. ) ;
#21903=CARTESIAN_POINT ( 'NONE',  ( -45.37157287525410254, -6.828427124746225374, 8.000000000000035527 ) ) ;
#21905=AXIS2_PLACEMENT_3D ( 'NONE', #5796, #11416, #20257 ) ;
#21907=CIRCLE ( 'NONE', #22668, 6.700000000000039257 ) ;
#21915=ADVANCED_FACE ( 'NONE', ( #9938 ), #18993, .T. ) ;
#21925=VECTOR ( 'NONE', #4451, 1000.000000000000227 ) ;
#21928=VERTEX_POINT ( 'NONE', #5227 ) ;
#21940=CARTESIAN_POINT ( 'NONE',  ( -6.000000000000074607, 7.999999999999958256, 7.500000000000062172 ) ) ;
#21952=VERTEX_POINT ( 'NONE', #1349 ) ;
#21959=EDGE_CURVE ( 'NONE', #1433, #21722, #5335, .T. ) ;
#21974=CIRCLE ( 'NONE', #20093, 3.500000000000023981 ) ;
#21976=CARTESIAN_POINT ( 'NONE',  ( -43.10883117545717624, 4.565685424949221805, 8.000000000000076383 ) ) ;
#21987=CARTESIAN_POINT ( 'NONE',  ( -89.70000000000064233, 5.551115123125782702E-14, -2.000000000000001776 ) ) ;
#21997=CARTESIAN_POINT ( 'NONE',  ( -53.99613665484950786, 2.700000000000021938, -13.19342998475048212 ) ) ;
#22006=FACE_OUTER_BOUND ( 'NONE', #6757, .T. ) ;
#22013=FACE_OUTER_BOUND ( 'NONE', #13949, .T. ) ;
#22014=EDGE_CURVE ( 'NONE', #6243, #8200, #12257, .T. ) ;
#22027=ORIENTED_EDGE ( 'NONE', *, *, #23171, .T. ) ;
#22028=ORIENTED_EDGE ( 'NONE', *, *, #19313, .T. ) ;
#22030=ORIENTED_EDGE ( 'NONE', *, *, #16826, .T. ) ;
#22036=EDGE_CURVE ( 'NONE', #8174, #4432, #11514, .T. ) ;
#22047=CARTESIAN_POINT ( 'NONE',  ( -95.70000000000058549, -0.5000000000000975886, 1.000000000000014655 ) ) ;
#22054=CARTESIAN_POINT ( 'NONE',  ( -64.00000000000045475, 6.245004513516505540E-14, -1.999999999999974021 ) ) ;
#22059=PRODUCT_DEFINITION_CONTEXT ( 'detailed design', #19916, 'design' ) ;
#22061=FACE_OUTER_BOUND ( 'NONE', #3526, .T. ) ;
#22062=EDGE_LOOP ( 'NONE', ( #7454, #4866, #899, #8551 ) ) ;
#22064=CIRCLE ( 'NONE', #14533, 2.000000000000015543 ) ;
#22068=ORIENTED_EDGE ( 'NONE', *, *, #19004, .T. ) ;
#22073=DIRECTION ( 'NONE',  ( -0.7071067811865534569, -0.7071067811865416886, -1.565905175853764455E-16 ) ) ;
#22078=ADVANCED_FACE ( 'NONE', ( #7222 ), #19922, .T. ) ;
#22080=AXIS2_PLACEMENT_3D ( 'NONE', #17710, #10427, #9014 ) ;
#22084=VECTOR ( 'NONE', #4444, 1000.000000000000114 ) ;
#22086=EDGE_CURVE ( 'NONE', #5438, #22523, #22064, .T. ) ;
#22087=AXIS2_PLACEMENT_3D ( 'NONE', #12285, #21490, #14069 ) ;
#22088=TOROIDAL_SURFACE ( 'NONE', #19076, 6.700000000000001066, 0.5000000000000000000 ) ;
#22089=DIRECTION ( 'NONE',  ( 1.000000000000000000, 1.110223024625164429E-16, -1.298062744027674633E-32 ) ) ;
#22091=ORIENTED_EDGE ( 'NONE', *, *, #8834, .F. ) ;
#22092=ORIENTED_EDGE ( 'NONE', *, *, #2034, .F. ) ;
#22097=AXIS2_PLACEMENT_3D ( 'NONE', #18807, #2680, #11617 ) ;
#22098=CYLINDRICAL_SURFACE ( 'NONE', #852, 6.000000000000037303 ) ;
#22100=CARTESIAN_POINT ( 'NONE',  ( -50.65685424949277404, -0.5000000000001045830, -7.500000000000062172 ) ) ;
#22102=CIRCLE ( 'NONE', #1428, 0.5000000000000029976 ) ;
#22115=AXIS2_PLACEMENT_3D ( 'NONE', #4943, #2963, #5306 ) ;
#22119=EDGE_LOOP ( 'NONE', ( #1015, #6886, #3023, #8244 ) ) ;
#22123=CARTESIAN_POINT ( 'NONE',  ( -6.000000000000074607, 7.499999999999958256, 7.500000000000062172 ) ) ;
#22129=CARTESIAN_POINT ( 'NONE',  ( -50.65685424949281668, 2.700000000000021938, -7.500000000000089706 ) ) ;
#22149=VERTEX_POINT ( 'NONE', #2607 ) ;
#22158=ADVANCED_FACE ( 'NONE', ( #22255 ), #851, .T. ) ;
#22159=AXIS2_PLACEMENT_3D ( 'NONE', #1470, #8645, #15802 ) ;
#22163=EDGE_CURVE ( 'NONE', #5689, #8200, #6263, .T. ) ;
#22166=DIRECTION ( 'NONE',  ( -2.013525853228507892E-32, -6.902532920683810383E-31, 1.000000000000000000 ) ) ;
#22174=EDGE_CURVE ( 'NONE', #278, #6998, #15418, .T. ) ;
#22181=ORIENTED_EDGE ( 'NONE', *, *, #21858, .T. ) ;
#22183=ORIENTED_EDGE ( 'NONE', *, *, #8263, .T. ) ;
#22184=DIRECTION ( 'NONE',  ( 2.013525853228507892E-32, 6.902532920683810383E-31, -1.000000000000000000 ) ) ;
#22189=DIRECTION ( 'NONE',  ( -2.710505431213791653E-16, -1.000000000000000000, 4.807121141190541565E-31 ) ) ;
#22192=AXIS2_PLACEMENT_3D ( 'NONE', #19676, #12016, #17432 ) ;
#22197=EDGE_CURVE ( 'NONE', #21644, #5438, #8156, .T. ) ;
#22199=EDGE_CURVE ( 'NONE', #19105, #22821, #1030, .T. ) ;
#22204=DIRECTION ( 'NONE',  ( 0.7071067811865490160, 0.7071067811865460184, 1.565905175853767167E-16 ) ) ;
#22208=VECTOR ( 'NONE', #15984, 1000.000000000000000 ) ;
#22212=ORIENTED_EDGE ( 'NONE', *, *, #22898, .F. ) ;
#22213=DIRECTION ( 'NONE',  ( 2.859620781426167795E-30, 1.000000000000000000, -7.806255641895663479E-15 ) ) ;
#22219=CARTESIAN_POINT ( 'NONE',  ( -45.01801948466091829, 6.474873734152897242, 7.500000000000034639 ) ) ;
#22222=CYLINDRICAL_SURFACE ( 'NONE', #16558, 10.00000000000006395 ) ;
#22223=DIRECTION ( 'NONE',  ( -1.000000000000000000, 1.550910762415526064E-16, 0.000000000000000000 ) ) ;
#22224=DIRECTION ( 'NONE',  ( 0.1556420233463076119, 0.000000000000000000, 0.9878135252003121813 ) ) ;
#22235=ORIENTED_EDGE ( 'NONE', *, *, #16818, .T. ) ;
#22255=FACE_OUTER_BOUND ( 'NONE', #5666, .T. ) ;
#22258=VERTEX_POINT ( 'NONE', #18613 ) ;
#22264=ORIENTED_EDGE ( 'NONE', *, *, #14555, .F. ) ;
#22273=FACE_OUTER_BOUND ( 'NONE', #8176, .T. ) ;
#22274=AXIS2_PLACEMENT_3D ( 'NONE', #21479, #17577, #8761 ) ;
#22275=CARTESIAN_POINT ( 'NONE',  ( -90.63385214007838897, -0.5000000000000628386, -7.926881151201908615 ) ) ;
#22281=CARTESIAN_POINT ( 'NONE',  ( -55.05572809000123868, -0.5000000000001045830, -7.500000000000062172 ) ) ;
#22286=LINE ( 'NONE', #4746, #20218 ) ;
#22287=LINE ( 'NONE', #1001, #13782 ) ;
#22296=CIRCLE ( 'NONE', #22671, 0.5000000000000004441 ) ;
#22314=CIRCLE ( 'NONE', #7291, 9.500000000000049738 ) ;
#22319=FACE_OUTER_BOUND ( 'NONE', #7088, .T. ) ;
#22331=AXIS2_PLACEMENT_3D ( 'NONE', #23125, #16035, #12039 ) ;
#22332=ORIENTED_EDGE ( 'NONE', *, *, #14867, .F. ) ;
#22333=CARTESIAN_POINT ( 'NONE',  ( -2.700000000000091216, -2.000000000000043521, 7.500000000000034639 ) ) ;
#22335=ORIENTED_EDGE ( 'NONE', *, *, #2396, .F. ) ;
#22341=ADVANCED_FACE ( 'NONE', ( #1964 ), #16320, .T. ) ;
#22345=FACE_OUTER_BOUND ( 'NONE', #6248, .T. ) ;
#22348=AXIS2_PLACEMENT_3D ( 'NONE', #19991, #3984, #21876 ) ;
#22356=CARTESIAN_POINT ( 'NONE',  ( -89.70000000000059970, 3.200000000000057021, 1.000000000000000888 ) ) ;
#22378=VECTOR ( 'NONE', #2005, 1000.000000000000114 ) ;
#22396=DIRECTION ( 'NONE',  ( 1.000000000000000000, 0.000000000000000000, 0.000000000000000000 ) ) ;
#22397=DIRECTION ( 'NONE',  ( 1.000000000000000000, 1.479114197289387852E-30, -2.013525853228518840E-32 ) ) ;
#22400=DIRECTION ( 'NONE',  ( -1.000000000000000000, -2.220446049250313081E-16, 0.000000000000000000 ) ) ;
#22404=LINE ( 'NONE', #6058, #12649 ) ;
#22405=ORIENTED_EDGE ( 'NONE', *, *, #8695, .F. ) ;
#22407=ORIENTED_EDGE ( 'NONE', *, *, #17293, .T. ) ;
#22412=ORIENTED_EDGE ( 'NONE', *, *, #20035, .F. ) ;
#22414=ADVANCED_FACE ( 'NONE', ( #4084 ), #11260, .F. ) ;
#22415=VERTEX_POINT ( 'NONE', #11025 ) ;
#22419=EDGE_LOOP ( 'NONE', ( #17093, #21210, #7760, #21617 ) ) ;
#22420=CARTESIAN_POINT ( 'NONE',  ( -55.25320565519150051, 9.020562075079396891E-14, 7.500000000000062172 ) ) ;
#22426=DIRECTION ( 'NONE',  ( 1.000000000000000000, -9.957992501029406452E-17, -2.655250634480538332E-32 ) ) ;
#22427=TOROIDAL_SURFACE ( 'NONE', #13779, 2.500000000000002220, 0.5000000000000000000 ) ;
#22433=CARTESIAN_POINT ( 'NONE',  ( -3.200000000000105427, 1.999999999999911626, -7.500000000000062172 ) ) ;
#22437=AXIS2_PLACEMENT_3D ( 'NONE', #4452, #22813, #8228 ) ;
#22438=ORIENTED_EDGE ( 'NONE', *, *, #14695, .F. ) ;
#22442=DIRECTION ( 'NONE',  ( -0.9878135252003127365, -2.193386639427060722E-16, 0.1556420233463029767 ) ) ;
#22443=DIRECTION ( 'NONE',  ( -1.000000000000000000, 1.626303258728243832E-16, -1.778091562876213388E-14 ) ) ;
#22445=AXIS2_PLACEMENT_3D ( 'NONE', #13398, #11167, #3985 ) ;
#22447=FACE_OUTER_BOUND ( 'NONE', #8576, .T. ) ;
#22453=ADVANCED_FACE ( 'NONE', ( #12792 ), #13059, .T. ) ;
#22466=VECTOR ( 'NONE', #13519, 1000.000000000000000 ) ;
#22482=DIRECTION ( 'NONE',  ( 0.9706398123736330597, -1.505375731439247434E-16, 0.2405376366294442736 ) ) ;
#22486=DIRECTION ( 'NONE',  ( 0.000000000000000000, 0.000000000000000000, -1.000000000000000000 ) ) ;
#22488=ADVANCED_FACE ( 'NONE', ( #16890 ), #6660, .T. ) ;
#22493=CARTESIAN_POINT ( 'NONE',  ( -95.70000000000069917, 0.5000000000000073275, -2.000000000000001776 ) ) ;
#22494=AXIS2_PLACEMENT_3D ( 'NONE', #6051, #1925, #5938 ) ;
#22496=DIRECTION ( 'NONE',  ( 0.000000000000000000, -1.000000000000000000, 0.000000000000000000 ) ) ;
#22500=EDGE_LOOP ( 'NONE', ( #7375, #8696, #5055, #17414 ) ) ;
#22505=ORIENTED_EDGE ( 'NONE', *, *, #196, .F. ) ;
#22509=CYLINDRICAL_SURFACE ( 'NONE', #6583, 0.5000000000000035527 ) ;
#22512=CYLINDRICAL_SURFACE ( 'NONE', #8895, 2.800000000000000266 ) ;
#22514=CARTESIAN_POINT ( 'NONE',  ( -45.01801948466091829, 6.474873734152938987, -7.500000000000062172 ) ) ;
#22517=DIRECTION ( 'NONE',  ( 1.550910762415566494E-16, 1.000000000000000000, -8.135128085091684243E-31 ) ) ;
#22523=VERTEX_POINT ( 'NONE', #1151 ) ;
#22530=ORIENTED_EDGE ( 'NONE', *, *, #21604, .T. ) ;
#22531=AXIS2_PLACEMENT_3D ( 'NONE', #14572, #12692, #7299 ) ;
#22532=VERTEX_POINT ( 'NONE', #22676 ) ;
#22539=ORIENTED_EDGE ( 'NONE', *, *, #3757, .F. ) ;
#22545=CARTESIAN_POINT ( 'NONE',  ( -45.01801948466092540, 6.474873734152931881, -8.000000000000062172 ) ) ;
#22548=LINE ( 'NONE', #15358, #5988 ) ;
#22549=TOROIDAL_SURFACE ( 'NONE', #16885, 9.499999999999998224, 0.5000000000000000000 ) ;
#22551=CARTESIAN_POINT ( 'NONE',  ( -6.000000000000116351, 4.799999999999957190, -7.500000000000062172 ) ) ;
#22558=VERTEX_POINT ( 'NONE', #8082 ) ;
#22560=DIRECTION ( 'NONE',  ( 1.000000000000000000, -1.550910762415513985E-16, -3.012982189080959477E-32 ) ) ;
#22564=FACE_OUTER_BOUND ( 'NONE', #19009, .T. ) ;
#22572=CARTESIAN_POINT ( 'NONE',  ( -87.15000000000055991, -9.060110299520993284E-14, -2.000000000000002220 ) ) ;
#22573=DIRECTION ( 'NONE',  ( 1.550910762415566494E-16, 1.000000000000000000, -8.135128085091684243E-31 ) ) ;
#22597=DIRECTION ( 'NONE',  ( 2.013525853228507892E-32, 6.902532920683810383E-31, -1.000000000000000000 ) ) ;
#22599=DIRECTION ( 'NONE',  ( 1.000000000000000000, -2.633062418893351796E-15, 0.000000000000000000 ) ) ;
#22602=CARTESIAN_POINT ( 'NONE',  ( -42.54314575050782565, -4.800000000000064659, -8.000000000000007105 ) ) ;
#22603=ORIENTED_EDGE ( 'NONE', *, *, #17293, .F. ) ;
#22607=CIRCLE ( 'NONE', #10938, 0.5000000000000029976 ) ;
#22609=ORIENTED_EDGE ( 'NONE', *, *, #13004, .F. ) ;
#22619=LINE ( 'NONE', #12135, #9246 ) ;
#22624=EDGE_CURVE ( 'NONE', #1329, #15019, #14189, .T. ) ;
#22626=CARTESIAN_POINT ( 'NONE',  ( -8.326672684688674053E-14, -2.000000000000029310, 8.000000000000076383 ) ) ;
#22628=VECTOR ( 'NONE', #22073, 1000.000000000000000 ) ;
#22635=EDGE_CURVE ( 'NONE', #4139, #7855, #7059, .T. ) ;
#22638=ORIENTED_EDGE ( 'NONE', *, *, #13748, .T. ) ;
#22642=EDGE_CURVE ( 'NONE', #13378, #4065, #1599, .T. ) ;
#22668=AXIS2_PLACEMENT_3D ( 'NONE', #19706, #14409, #10976 ) ;
#22671=AXIS2_PLACEMENT_3D ( 'NONE', #6857, #1684, #17313 ) ;
#22676=CARTESIAN_POINT ( 'NONE',  ( -50.65685424949281668, 3.200000000000022382, 7.500000000000034639 ) ) ;
#22678=ADVANCED_FACE ( 'NONE', ( #19727 ), #2917, .T. ) ;
#22679=ORIENTED_EDGE ( 'NONE', *, *, #19894, .F. ) ;
#22684=CARTESIAN_POINT ( 'NONE',  ( -67.28510754798017501, -1.040834085586084257E-13, 12.22107821754960000 ) ) ;
#22686=ORIENTED_EDGE ( 'NONE', *, *, #13997, .T. ) ;
#22687=AXIS2_PLACEMENT_3D ( 'NONE', #15034, #11738, #22223 ) ;
#22695=FACE_OUTER_BOUND ( 'NONE', #13869, .T. ) ;
#22697=DIRECTION ( 'NONE',  ( -2.013525853228507892E-32, -6.902532920683810383E-31, 1.000000000000000000 ) ) ;
#22702=DIRECTION ( 'NONE',  ( -2.013525853228507892E-32, -6.902532920683810383E-31, 1.000000000000000000 ) ) ;
#22705=CIRCLE ( 'NONE', #22331, 0.5000000000000028866 ) ;
#22711=EDGE_CURVE ( 'NONE', #4165, #4144, #17568, .T. ) ;
#22716=AXIS2_PLACEMENT_3D ( 'NONE', #1763, #19650, #21660 ) ;
#22717=DIRECTION ( 'NONE',  ( 0.7071067811865507924, 0.7071067811865441310, 2.121016688166342479E-16 ) ) ;
#22720=DIRECTION ( 'NONE',  ( 1.000000000000000000, -1.424116703980815236E-16, -2.931272055834072749E-32 ) ) ;
#22721=FACE_OUTER_BOUND ( 'NONE', #16945, .T. ) ;
#22723=DIRECTION ( 'NONE',  ( 2.013525853228507892E-32, 6.902532920683810383E-31, -1.000000000000000000 ) ) ;
#22727=AXIS2_PLACEMENT_3D ( 'NONE', #7306, #15866, #14473 ) ;
#22733=ORIENTED_EDGE ( 'NONE', *, *, #5664, .F. ) ;
#22738=LINE ( 'NONE', #4954, #5397 ) ;
#22742=DIRECTION ( 'NONE',  ( -2.013525853228507892E-32, -6.902532920683810383E-31, 1.000000000000000000 ) ) ;
#22747=CARTESIAN_POINT ( 'NONE',  ( -64.00000000000045475, 6.245004513516505540E-14, -1.999999999999974021 ) ) ;
#22750=CARTESIAN_POINT ( 'NONE',  ( -89.70000000000055707, -3.200000000000091660, -1.999999999999946265 ) ) ;
#22757=ORIENTED_EDGE ( 'NONE', *, *, #7975, .F. ) ;
#22775=CARTESIAN_POINT ( 'NONE',  ( -55.05572809000126711, 2.700000000000021938, -7.500000000000034639 ) ) ;
#22790=EDGE_CURVE ( 'NONE', #16175, #19930, #22286, .T. ) ;
#22791=VECTOR ( 'NONE', #416, 1000.000000000000000 ) ;
#22801=VERTEX_POINT ( 'NONE', #15446 ) ;
#22813=DIRECTION ( 'NONE',  ( -0.9878135252003120703, -1.331202777560448839E-30, 0.1556420233463080560 ) ) ;
#22820=CIRCLE ( 'NONE', #14172, 1.300000000000009592 ) ;
#22821=VERTEX_POINT ( 'NONE', #8288 ) ;
#22822=ORIENTED_EDGE ( 'NONE', *, *, #20091, .T. ) ;
#22824=EDGE_CURVE ( 'NONE', #19389, #2652, #14210, .T. ) ;
#22827=FACE_OUTER_BOUND ( 'NONE', #544, .T. ) ;
#22831=LINE ( 'NONE', #20718, #12346 ) ;
#22836=CARTESIAN_POINT ( 'NONE',  ( -0.5000000000000975886, 1.999999999999932498, -7.500000000000007105 ) ) ;
#22840=CARTESIAN_POINT ( 'NONE',  ( -45.56568542494959928, -0.5000000000000698330, -8.000000000000035527 ) ) ;
#22850=EDGE_LOOP ( 'NONE', ( #1998, #17630, #11629, #9168 ) ) ;
#22859=AXIS2_PLACEMENT_3D ( 'NONE', #14442, #21158, #99 ) ;
#22864=DIRECTION ( 'NONE',  ( -1.000000000000000000, -2.220446049250297797E-16, 0.000000000000000000 ) ) ;
#22868=CARTESIAN_POINT ( 'NONE',  ( -42.54314575050799618, 3.999999999999996447, 8.000000000000035527 ) ) ;
#22877=EDGE_LOOP ( 'NONE', ( #10959, #13627, #3362, #9044 ) ) ;
#22879=AXIS2_PLACEMENT_3D ( 'NONE', #5280, #12323, #7285 ) ;
#22885=ORIENTED_EDGE ( 'NONE', *, *, #17990, .F. ) ;
#22887=ORIENTED_EDGE ( 'NONE', *, *, #3938, .F. ) ;
#22888=CARTESIAN_POINT ( 'NONE',  ( -42.54314575050793934, 7.999999999999992895, 8.000000000000035527 ) ) ;
#22889=DIRECTION ( 'NONE',  ( -1.000000000000000000, 0.000000000000000000, 0.000000000000000000 ) ) ;
#22890=ORIENTED_EDGE ( 'NONE', *, *, #13863, .F. ) ;
#22896=DIRECTION ( 'NONE',  ( 1.000000000000000000, 2.220446049250314560E-16, 0.000000000000000000 ) ) ;
#22898=EDGE_CURVE ( 'NONE', #8200, #19103, #13449, .T. ) ;
#22903=DIRECTION ( 'NONE',  ( 0.000000000000000000, 1.000000000000000000, 0.000000000000000000 ) ) ;
#22909=VERTEX_POINT ( 'NONE', #23232 ) ;
#22918=CARTESIAN_POINT ( 'NONE',  ( -45.37157287525410254, -6.828427124746218269, 8.000000000000035527 ) ) ;
#22923=CYLINDRICAL_SURFACE ( 'NONE', #22097, 0.5000000000000004441 ) ;
#22926=EDGE_CURVE ( 'NONE', #18025, #7684, #10072, .T. ) ;
#22936=DIRECTION ( 'NONE',  ( -2.220446049250313081E-16, 1.000000000000000000, -7.025792437124636392E-31 ) ) ;
#22937=VERTEX_POINT ( 'NONE', #19689 ) ;
#22951=DIRECTION ( 'NONE',  ( 0.000000000000000000, 1.000000000000000000, 0.000000000000000000 ) ) ;
#22955=LINE ( 'NONE', #17049, #5231 ) ;
#22959=DIRECTION ( 'NONE',  ( -0.7071067811865507924, -0.7071067811865444641, 1.064654809502291460E-15 ) ) ;
#22966=ORIENTED_EDGE ( 'NONE', *, *, #197, .T. ) ;
#22969=ORIENTED_EDGE ( 'NONE', *, *, #1757, .T. ) ;
#22972=CARTESIAN_POINT ( 'NONE',  ( -95.70000000000065654, -1.318389841742373392E-13, -2.000000000000029310 ) ) ;
#22980=CARTESIAN_POINT ( 'NONE',  ( -64.00000000000038369, -3.200000000000081446, -2.000000000000029310 ) ) ;
#22982=DIRECTION ( 'NONE',  ( 0.7071067811865507924, 0.7071067811865444641, -1.064654809502291460E-15 ) ) ;
#22985=CARTESIAN_POINT ( 'NONE',  ( -42.54314575050793934, 7.499999999999992895, 7.500000000000062172 ) ) ;
#22987=AXIS2_PLACEMENT_3D ( 'NONE', #15587, #2890, #13830 ) ;
#22988=VECTOR ( 'NONE', #12926, 1000.000000000000227 ) ;
#22991=EDGE_LOOP ( 'NONE', ( #19952, #21361, #22887, #13333 ) ) ;
#22996=VERTEX_POINT ( 'NONE', #391 ) ;
#22997=EDGE_LOOP ( 'NONE', ( #92, #16801, #15714, #20706 ) ) ;
#23001=DIRECTION ( 'NONE',  ( -0.9878135252003126254, 5.551115123125605208E-17, 0.1556420233463029767 ) ) ;
#23011=DIRECTION ( 'NONE',  ( -0.7071067811865454633, 0.7071067811865497932, 0.000000000000000000 ) ) ;
#23017=DIRECTION ( 'NONE',  ( -1.000000000000000000, -1.479114197289387852E-30, 2.013525853228518840E-32 ) ) ;
#23021=EDGE_LOOP ( 'NONE', ( #11825, #11120, #395, #19902 ) ) ;
#23028=VERTEX_POINT ( 'NONE', #13084 ) ;
#23040=FACE_OUTER_BOUND ( 'NONE', #6908, .T. ) ;
#23041=CARTESIAN_POINT ( 'NONE',  ( -95.20000000000065654, 3.200000000000015277, -2.000000000000001776 ) ) ;
#23042=CIRCLE ( 'NONE', #2736, 0.5000000000000038858 ) ;
#23045=DIRECTION ( 'NONE',  ( 2.220446049250313081E-16, -1.000000000000000000, 7.025792437124636392E-31 ) ) ;
#23046=DIRECTION ( 'NONE',  ( -1.000000000000000000, 0.000000000000000000, 0.000000000000000000 ) ) ;
#23047=EDGE_CURVE ( 'NONE', #9172, #2421, #16066, .T. ) ;
#23066=VERTEX_POINT ( 'NONE', #7337 ) ;
#23086=EDGE_CURVE ( 'NONE', #21118, #10966, #18383, .T. ) ;
#23089=EDGE_LOOP ( 'NONE', ( #17098, #1702, #19350, #3001 ) ) ;
#23091=ORIENTED_EDGE ( 'NONE', *, *, #1182, .T. ) ;
#23093=EDGE_LOOP ( 'NONE', ( #7344, #10771, #781, #2144 ) ) ;
#23097=DIRECTION ( 'NONE',  ( -1.000000000000000000, -1.479114197289388027E-30, 2.013525853228518840E-32 ) ) ;
#23101=CARTESIAN_POINT ( 'NONE',  ( -67.40537636629485974, -2.700000000000125855, 12.70639812373639010 ) ) ;
#23105=DIRECTION ( 'NONE',  ( 0.7071067811865506814, -0.7071067811865445751, 6.116169571546738730E-15 ) ) ;
#23125=CARTESIAN_POINT ( 'NONE',  ( -91.02295700146254376, -0.5000000000001045830, 6.338518968055040226 ) ) ;
#23137=ADVANCED_FACE ( 'NONE', ( #972 ), #13550, .T. ) ;
#23141=CARTESIAN_POINT ( 'NONE',  ( -50.65685424949280247, -1.040834085586084257E-13, 7.500000000000062172 ) ) ;
#23145=CIRCLE ( 'NONE', #15998, 2.550000000000010481 ) ;
#23151=ORIENTED_EDGE ( 'NONE', *, *, #8934, .T. ) ;
#23152=ORIENTED_EDGE ( 'NONE', *, *, #20317, .T. ) ;
#23161=CARTESIAN_POINT ( 'NONE',  ( -6.000000000000130562, 1.999999999999960032, -8.000000000000035527 ) ) ;
#23165=DIRECTION ( 'NONE',  ( -1.000000000000000000, 0.000000000000000000, 0.000000000000000000 ) ) ;
#23171=EDGE_CURVE ( 'NONE', #16292, #1099, #13321, .T. ) ;
#23178=EDGE_LOOP ( 'NONE', ( #19953, #17417, #8699, #19598 ) ) ;
#23187=CARTESIAN_POINT ( 'NONE',  ( -67.28510754798028870, 3.200000000000022382, 12.22107821754958579 ) ) ;
#23188=CARTESIAN_POINT ( 'NONE',  ( -42.54314575050796776, 3.999999999999996447, -8.000000000000035527 ) ) ;
#23193=LINE ( 'NONE', #21197, #3498 ) ;
#23197=VECTOR ( 'NONE', #3331, 1000.000000000000227 ) ;
#23210=EDGE_CURVE ( 'NONE', #21722, #6874, #17212, .T. ) ;
#23212=LINE ( 'NONE', #22972, #15149 ) ;
#23217=VECTOR ( 'NONE', #17767, 1000.000000000000000 ) ;
#23220=AXIS2_PLACEMENT_3D ( 'NONE', #14309, #21138, #10769 ) ;
#23221=CARTESIAN_POINT ( 'NONE',  ( -91.02295700146257218, -3.200000000000101874, 6.338518968055012692 ) ) ;
#23224=APPLICATION_CONTEXT ( 'automotive_design' ) ;
#23232=CARTESIAN_POINT ( 'NONE',  ( -6.000000000000019540, -8.000000000000042633, 7.500000000000062172 ) ) ;
#23236=AXIS2_PLACEMENT_3D ( 'NONE', #15960, #5276, #23165 ) ;
#23237=ORIENTED_EDGE ( 'NONE', *, *, #19604, .T. ) ;
#23241=ORIENTED_EDGE ( 'NONE', *, *, #11679, .T. ) ;
#23245=EDGE_LOOP ( 'NONE', ( #2671, #11183, #510, #14513 ) ) ;
#23257=DIRECTION ( 'NONE',  ( 2.220446049250313081E-16, -1.000000000000000000, 7.025792437124636392E-31 ) ) ;
#23261=ORIENTED_EDGE ( 'NONE', *, *, #15752, .T. ) ;
#23262=TOROIDAL_SURFACE ( 'NONE', #16087, 4.500000000000002665, 0.5000000000000000000 ) ;
#23266=ORIENTED_EDGE ( 'NONE', *, *, #16432, .T. ) ;
ENDSEC;
END-ISO-10303-21;
